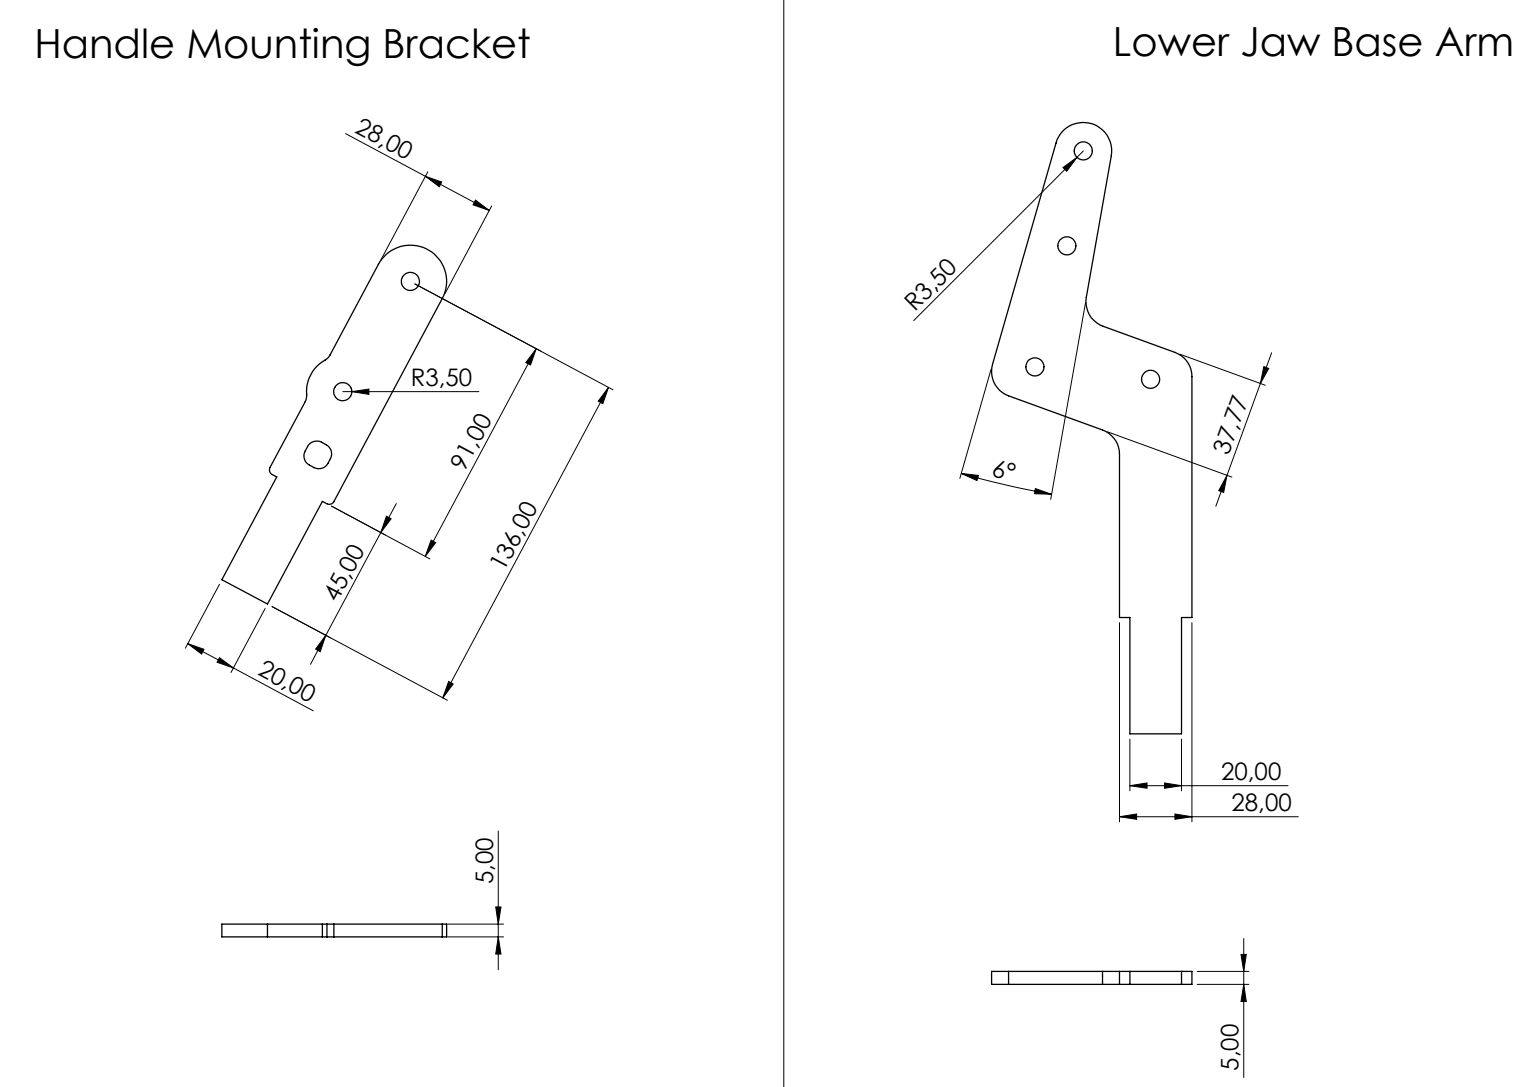
ISO-10303-21;
HEADER;
FILE_DESCRIPTION (('STEP AP214'),
    '1' );
FILE_NAME ('Lower Jaw Base Arm.step',
    '2026-10-06T08:24:18',
    ( '' ),
    ( '' ),
    'SwSTEP 2.0',
    'SolidWorks 2020',
    '' );
FILE_SCHEMA (( 'AUTOMOTIVE_DESIGN' ));
ENDSEC;

DATA;
#13=LINE ( 'NONE', #6569, #9092 ) ;
#17=UNCERTAINTY_MEASURE_WITH_UNIT (LENGTH_MEASURE( 1.000000000000000082E-05 ), #9490, 'distance_accuracy_value', 'NONE');
#20=ORIENTED_EDGE ( 'NONE', *, *, #8443, .F. ) ;
#27=EDGE_CURVE ( 'NONE', #6443, #1984, #9042, .T. ) ;
#34=EDGE_LOOP ( 'NONE', ( #2547, #9848, #2016, #7759 ) ) ;
#35=DIRECTION ( 'NONE',  ( -1.000000000000000000, 0.000000000000000000, 0.000000000000000000 ) ) ;
#41=DIRECTION ( 'NONE',  ( 0.000000000000000000, 0.000000000000000000, 1.000000000000000000 ) ) ;
#87=AXIS2_PLACEMENT_3D ( 'NONE', #9230, #1862, #35 ) ;
#93=CARTESIAN_POINT ( 'NONE',  ( 7.420201433257000545, -2.500000000000000000, -419.8948508258000061 ) ) ;
#98=DIRECTION ( 'NONE',  ( -0.9848077530122131273, 0.000000000000000000, -0.1736481776669018817 ) ) ;
#110=EDGE_LOOP ( 'NONE', ( #3310, #285 ) ) ;
#113=EDGE_CURVE ( 'NONE', #8766, #6326, #6244, .T. ) ;
#114=EDGE_CURVE ( 'NONE', #1984, #5924, #1786, .T. ) ;
#144=DIRECTION ( 'NONE',  ( 0.000000000000000000, -1.000000000000000000, 0.000000000000000000 ) ) ;
#177=CARTESIAN_POINT ( 'NONE',  ( -26.82908671702000802, -2.500000000000000000, -441.1544246730000509 ) ) ;
#178=CARTESIAN_POINT ( 'NONE',  ( 14.00000000000000000, 2.500000000000000000, -410.4979246179000256 ) ) ;
#187=AXIS2_PLACEMENT_3D ( 'NONE', #7775, #1275, #419 ) ;
#215=VERTEX_POINT ( 'NONE', #8725 ) ;
#219=DIRECTION ( 'NONE',  ( 0.9848077530122130163, 0.000000000000000000, 0.1736481776669023813 ) ) ;
#223=VERTEX_POINT ( 'NONE', #5395 ) ;
#235=EDGE_CURVE ( 'NONE', #9158, #4552, #1974, .T. ) ;
#244=CARTESIAN_POINT ( 'NONE',  ( -26.82908671702000802, -2.500000000000000000, -441.1544246730000509 ) ) ;
#285=ORIENTED_EDGE ( 'NONE', *, *, #8827, .T. ) ;
#289=VERTEX_POINT ( 'NONE', #1316 ) ;
#303=APPLICATION_CONTEXT ( 'automotive_design' ) ;
#305=DIRECTION ( 'NONE',  ( 0.000000000000000000, 1.000000000000000000, 0.000000000000000000 ) ) ;
#308=LINE ( 'NONE', #2126, #3162 ) ;
#338=LINE ( 'NONE', #980, #680 ) ;
#339=ORIENTED_EDGE ( 'NONE', *, *, #9047, .F. ) ;
#344=VERTEX_POINT ( 'NONE', #2396 ) ;
#360=CIRCLE ( 'NONE', #7394, 3.500000000000000000 ) ;
#376=CARTESIAN_POINT ( 'NONE',  ( -63.11273421720001409, 2.500000000000000000, -415.2750182148000135 ) ) ;
#377=CYLINDRICAL_SURFACE ( 'NONE', #3349, 3.500000000000003109 ) ;
#378=PLANE ( 'NONE',  #9312 ) ;
#403=ORIENTED_EDGE ( 'NONE', *, *, #6734, .T. ) ;
#419=DIRECTION ( 'NONE',  ( -0.9612616959383174509, 0.000000000000000000, -0.2756373558170044369 ) ) ;
#438=ORIENTED_EDGE ( 'NONE', *, *, #6849, .T. ) ;
#440=DIRECTION ( 'NONE',  ( 1.000000000000000000, 0.000000000000000000, 0.000000000000000000 ) ) ;
#444=EDGE_CURVE ( 'NONE', #7016, #4872, #3088, .T. ) ;
#447=CARTESIAN_POINT ( 'NONE',  ( -5.500000000000000000, 2.500000000000000000, -409.5000000000000568 ) ) ;
#478=FACE_OUTER_BOUND ( 'NONE', #9284, .T. ) ;
#480=CIRCLE ( 'NONE', #7844, 3.500000000000003109 ) ;
#494=LINE ( 'NONE', #3762, #7350 ) ;
#502=EDGE_LOOP ( 'NONE', ( #7761, #10328 ) ) ;
#506=DIRECTION ( 'NONE',  ( 1.000000000000000000, 0.000000000000000000, 0.000000000000000000 ) ) ;
#507=EDGE_CURVE ( 'NONE', #6146, #7283, #8033, .T. ) ;
#522=FILL_AREA_STYLE_COLOUR ( '', #3538 ) ;
#537=LINE ( 'NONE', #9560, #754 ) ;
#544=FACE_OUTER_BOUND ( 'NONE', #612, .T. ) ;
#549=FILL_AREA_STYLE ('',( #8596 ) ) ;
#555=CIRCLE ( 'NONE', #7588, 3.499999999999999556 ) ;
#564=CARTESIAN_POINT ( 'NONE',  ( -14.00000000000000000, 2.500000000000000000, -380.4979246178999688 ) ) ;
#580=LINE ( 'NONE', #7938, #3620 ) ;
#588=CIRCLE ( 'NONE', #7964, 3.499999999999999556 ) ;
#608=FACE_OUTER_BOUND ( 'NONE', #8794, .T. ) ;
#610=DIRECTION ( 'NONE',  ( 1.000000000000000000, 0.000000000000000000, 0.000000000000000000 ) ) ;
#612=EDGE_LOOP ( 'NONE', ( #2471, #339, #8409, #673 ) ) ;
#615=FACE_OUTER_BOUND ( 'NONE', #9397, .T. ) ;
#617=DIRECTION ( 'NONE',  ( -0.9396926207858973257, 0.000000000000000000, -0.3420201433256991330 ) ) ;
#638=ORIENTED_EDGE ( 'NONE', *, *, #1595, .F. ) ;
#657=FACE_OUTER_BOUND ( 'NONE', #6357, .T. ) ;
#658=DIRECTION ( 'NONE',  ( -1.000000000000000000, 0.000000000000000000, 0.000000000000000000 ) ) ;
#673=ORIENTED_EDGE ( 'NONE', *, *, #1413, .T. ) ;
#678=DIRECTION ( 'NONE',  ( 0.000000000000000000, 1.000000000000000000, 0.000000000000000000 ) ) ;
#680=VECTOR ( 'NONE', #1083, 1000.000000000000000 ) ;
#694=EDGE_CURVE ( 'NONE', #9461, #7519, #8991, .T. ) ;
#715=ORIENTED_EDGE ( 'NONE', *, *, #7705, .F. ) ;
#723=DIRECTION ( 'NONE',  ( 0.9848077530122130163, 0.000000000000000000, 0.1736481776669025201 ) ) ;
#731=VECTOR ( 'NONE', #6902, 1000.000000000000000 ) ;
#742=DIRECTION ( 'NONE',  ( 1.000000000000000000, 0.000000000000000000, 0.000000000000000000 ) ) ;
#754=VECTOR ( 'NONE', #1389, 1000.000000000000227 ) ;
#757=EDGE_CURVE ( 'NONE', #9634, #5121, #13, .T. ) ;
#758=DIRECTION ( 'NONE',  ( -1.000000000000000000, 0.000000000000000000, 0.000000000000000000 ) ) ;
#776=ORIENTED_EDGE ( 'NONE', *, *, #694, .F. ) ;
#816=VECTOR ( 'NONE', #6829, 1000.000000000000000 ) ;
#831=DIRECTION ( 'NONE',  ( 0.000000000000000000, -1.000000000000000000, 0.000000000000000000 ) ) ;
#853=CARTESIAN_POINT ( 'NONE',  ( 4.000000000000000000, -2.500000000000000000, -410.4979246179000256 ) ) ;
#865=VECTOR ( 'NONE', #3827, 1000.000000000000000 ) ;
#877=EDGE_LOOP ( 'NONE', ( #3684, #7845, #2714, #438 ) ) ;
#878=AXIS2_PLACEMENT_3D ( 'NONE', #2871, #7754, #8553 ) ;
#885=LINE ( 'NONE', #2614, #8061 ) ;
#886=VERTEX_POINT ( 'NONE', #9177 ) ;
#906=CARTESIAN_POINT ( 'NONE',  ( -28.01838671672000203, 2.500000000000000000, -497.7560445212000104 ) ) ;
#931=DIRECTION ( 'NONE',  ( -1.000000000000000000, 0.000000000000000000, 0.000000000000000000 ) ) ;
#940=AXIS2_PLACEMENT_3D ( 'NONE', #6757, #144, #6590 ) ;
#978=CARTESIAN_POINT ( 'NONE',  ( 14.00000000000000000, -2.500000000000000000, -410.4979246179000256 ) ) ;
#980=CARTESIAN_POINT ( 'NONE',  ( 14.00000000000000000, -2.500000000000000000, -317.5000000000000000 ) ) ;
#993=DIRECTION ( 'NONE',  ( 0.000000000000000000, -1.000000000000000000, 0.000000000000000000 ) ) ;
#995=FACE_OUTER_BOUND ( 'NONE', #6467, .T. ) ;
#997=EDGE_LOOP ( 'NONE', ( #6427, #6798, #10128, #4940 ) ) ;
#999=DIRECTION ( 'NONE',  ( 0.000000000000000000, -1.000000000000000000, 0.000000000000000000 ) ) ;
#1003=EDGE_CURVE ( 'NONE', #7519, #5811, #5243, .T. ) ;
#1024=EDGE_CURVE ( 'NONE', #5654, #10404, #308, .T. ) ;
#1027=DIRECTION ( 'NONE',  ( 0.1736481776669025201, 0.000000000000000000, -0.9848077530122130163 ) ) ;
#1031=DIRECTION ( 'NONE',  ( -1.000000000000000000, 0.000000000000000000, 0.000000000000000000 ) ) ;
#1047=DIRECTION ( 'NONE',  ( -0.9848077530122131273, 0.000000000000000000, -0.1736481776669018817 ) ) ;
#1049=CARTESIAN_POINT ( 'NONE',  ( 10.00000000000000000, -2.500000000000000000, -272.5000000000000000 ) ) ;
#1054=CARTESIAN_POINT ( 'NONE',  ( -10.00000000000000000, -2.500000000000000000, -317.5000000000000000 ) ) ;
#1065=DIRECTION ( 'NONE',  ( -0.2756373558170050475, 0.000000000000000000, 0.9612616959383172288 ) ) ;
#1079=DIRECTION ( 'NONE',  ( 0.000000000000000000, -1.000000000000000000, 0.000000000000000000 ) ) ;
#1083=DIRECTION ( 'NONE',  ( 0.000000000000000000, 1.000000000000000000, 0.000000000000000000 ) ) ;
#1084=EDGE_CURVE ( 'NONE', #6576, #215, #8309, .T. ) ;
#1103=ORIENTED_EDGE ( 'NONE', *, *, #7129, .T. ) ;
#1111=AXIS2_PLACEMENT_3D ( 'NONE', #8004, #8802, #4672 ) ;
#1143=CARTESIAN_POINT ( 'NONE',  ( 14.00000000000000000, -2.500000000000000000, -317.5000000000000000 ) ) ;
#1151=DIRECTION ( 'NONE',  ( 0.000000000000000000, 1.000000000000000000, 0.000000000000000000 ) ) ;
#1162=CIRCLE ( 'NONE', #3220, 11.00000000000000000 ) ;
#1175=LINE ( 'NONE', #8742, #10006 ) ;
#1185=DIRECTION ( 'NONE',  ( 0.9848077530122130163, 0.000000000000000000, 0.1736481776669023813 ) ) ;
#1188=EDGE_LOOP ( 'NONE', ( #2072, #8240, #8227, #5008 ) ) ;
#1194=AXIS2_PLACEMENT_3D ( 'NONE', #4119, #993, #6644 ) ;
#1201=ORIENTED_EDGE ( 'NONE', *, *, #1003, .T. ) ;
#1215=LINE ( 'NONE', #2785, #8659 ) ;
#1220=EDGE_LOOP ( 'NONE', ( #1727, #6254 ) ) ;
#1223=EDGE_CURVE ( 'NONE', #8790, #6146, #8438, .T. ) ;
#1229=LINE ( 'NONE', #6992, #2985 ) ;
#1233=AXIS2_PLACEMENT_3D ( 'NONE', #8007, #6501, #4787 ) ;
#1239=ADVANCED_FACE ( 'NONE', ( #4414 ), #6790, .T. ) ;
#1245=DIRECTION ( 'NONE',  ( 0.000000000000000000, 1.000000000000000000, 0.000000000000000000 ) ) ;
#1262=CARTESIAN_POINT ( 'NONE',  ( -37.87192209818999800, 2.500000000000000000, -461.0868123482000556 ) ) ;
#1273=ORIENTED_EDGE ( 'NONE', *, *, #1410, .F. ) ;
#1275=DIRECTION ( 'NONE',  ( 0.000000000000000000, 1.000000000000000000, 0.000000000000000000 ) ) ;
#1277=ADVANCED_FACE ( 'NONE', ( #8390, #4462, #9365, #4264, #6943 ), #4313, .F. ) ;
#1285=CARTESIAN_POINT ( 'NONE',  ( 4.000000000000000000, 2.656480000000000175, -410.4979246179000256 ) ) ;
#1290=CARTESIAN_POINT ( 'NONE',  ( 7.420201433257000545, 2.500000000000000000, -419.8948508258000061 ) ) ;
#1299=SURFACE_STYLE_USAGE ( .BOTH. , #10379 ) ;
#1316=CARTESIAN_POINT ( 'NONE',  ( 14.00000000000000000, 2.500000000000000000, -317.5000000000000000 ) ) ;
#1322=VERTEX_POINT ( 'NONE', #178 ) ;
#1324=AXIS2_PLACEMENT_3D ( 'NONE', #4265, #1079, #7534 ) ;
#1358=PLANE ( 'NONE',  #3824 ) ;
#1359=EDGE_LOOP ( 'NONE', ( #1930, #10581, #4963, #3339 ) ) ;
#1381=COLOUR_RGB ( '', 0.09019608, 0.27058824, 0.51372549) ;
#1385=DIRECTION ( 'NONE',  ( 0.000000000000000000, 1.000000000000000000, 0.000000000000000000 ) ) ;
#1389=DIRECTION ( 'NONE',  ( 0.9396926207858972147, 0.000000000000000000, 0.3420201433256990775 ) ) ;
#1405=PRESENTATION_STYLE_ASSIGNMENT (( #1299 ) ) ;
#1410=EDGE_CURVE ( 'NONE', #1779, #9634, #8644, .T. ) ;
#1413=EDGE_CURVE ( 'NONE', #9766, #8632, #588, .T. ) ;
#1437=ORIENTED_EDGE ( 'NONE', *, *, #3941, .F. ) ;
#1447=ORIENTED_EDGE ( 'NONE', *, *, #3836, .F. ) ;
#1465=DIRECTION ( 'NONE',  ( 0.000000000000000000, -1.000000000000000000, 0.000000000000000000 ) ) ;
#1474=DIRECTION ( 'NONE',  ( 0.000000000000000000, 0.000000000000000000, -1.000000000000000000 ) ) ;
#1479=ORIENTED_EDGE ( 'NONE', *, *, #6849, .F. ) ;
#1496=FACE_OUTER_BOUND ( 'NONE', #9347, .T. ) ;
#1510=VECTOR ( 'NONE', #8979, 1000.000000000000000 ) ;
#1511=LINE ( 'NONE', #4035, #8370 ) ;
#1517=CYLINDRICAL_SURFACE ( 'NONE', #2762, 3.499999999999999556 ) ;
#1529=LINE ( 'NONE', #564, #1934 ) ;
#1533=CARTESIAN_POINT ( 'NONE',  ( -30.87192209819000155, 2.500000000000000000, -461.0868123482000556 ) ) ;
#1539=VECTOR ( 'NONE', #4099, 1000.000000000000000 ) ;
#1554=CARTESIAN_POINT ( 'NONE',  ( -20.57979856674000629, -2.500000000000000000, -389.8948508258000061 ) ) ;
#1572=CARTESIAN_POINT ( 'NONE',  ( 14.00000000000000000, 2.500000000000000000, -410.4979246179000256 ) ) ;
#1595=EDGE_CURVE ( 'NONE', #5654, #6416, #2475, .T. ) ;
#1615=ORIENTED_EDGE ( 'NONE', *, *, #1024, .T. ) ;
#1621=CIRCLE ( 'NONE', #7626, 3.499999999999999556 ) ;
#1647=EDGE_LOOP ( 'NONE', ( #8599, #7824, #2420, #5607 ) ) ;
#1650=ORIENTED_EDGE ( 'NONE', *, *, #2610, .F. ) ;
#1654=DIRECTION ( 'NONE',  ( 0.000000000000000000, -1.000000000000000000, 0.000000000000000000 ) ) ;
#1667=ADVANCED_FACE ( 'NONE', ( #2269 ), #5535, .T. ) ;
#1673=CARTESIAN_POINT ( 'NONE',  ( -20.57979856674000629, 2.500000000000000000, -389.8948508258000061 ) ) ;
#1684=AXIS2_PLACEMENT_3D ( 'NONE', #10257, #2846, #2193 ) ;
#1695=MANIFOLD_SOLID_BREP ( 'Stock-MAS-686-1', #6776 ) ;
#1707=CYLINDRICAL_SURFACE ( 'NONE', #5477, 10.00000000000000000 ) ;
#1727=ORIENTED_EDGE ( 'NONE', *, *, #8494, .F. ) ;
#1736=DIRECTION ( 'NONE',  ( 0.000000000000000000, -1.000000000000000000, 0.000000000000000000 ) ) ;
#1747=CARTESIAN_POINT ( 'NONE',  ( -37.87192209818999800, -2.500000000000000000, -461.0868123482000556 ) ) ;
#1752=EDGE_CURVE ( 'NONE', #1322, #1779, #6013, .T. ) ;
#1764=LINE ( 'NONE', #5952, #10510 ) ;
#1779=VERTEX_POINT ( 'NONE', #5592 ) ;
#1786=LINE ( 'NONE', #5056, #7970 ) ;
#1801=ADVANCED_FACE ( 'NONE', ( #8069 ), #1517, .F. ) ;
#1807=EDGE_CURVE ( 'NONE', #6443, #6958, #3284, .T. ) ;
#1827=EDGE_LOOP ( 'NONE', ( #5391, #2707, #3495, #4698 ) ) ;
#1853=ORIENTED_EDGE ( 'NONE', *, *, #2590, .F. ) ;
#1862=DIRECTION ( 'NONE',  ( 0.000000000000000000, -1.000000000000000000, 0.000000000000000000 ) ) ;
#1872=DIRECTION ( 'NONE',  ( 0.000000000000000000, 1.000000000000000000, 0.000000000000000000 ) ) ;
#1891=EDGE_CURVE ( 'NONE', #1322, #2247, #9793, .T. ) ;
#1901=AXIS2_PLACEMENT_3D ( 'NONE', #2432, #3345, #5855 ) ;
#1903=ORIENTED_EDGE ( 'NONE', *, *, #444, .T. ) ;
#1918=LINE ( 'NONE', #1054, #6408 ) ;
#1924=PRODUCT ( 'Lower Jaw Base Arm', 'Lower Jaw Base Arm', '', ( #5587 ) ) ;
#1930=ORIENTED_EDGE ( 'NONE', *, *, #3836, .T. ) ;
#1934=VECTOR ( 'NONE', #3840, 1000.000000000000000 ) ;
#1940=EDGE_CURVE ( 'NONE', #223, #8573, #5502, .T. ) ;
#1973=DIRECTION ( 'NONE',  ( 0.000000000000000000, -1.000000000000000000, 0.000000000000000000 ) ) ;
#1974=LINE ( 'NONE', #1262, #10038 ) ;
#1976=CIRCLE ( 'NONE', #6248, 3.500000000000003109 ) ;
#1982=CARTESIAN_POINT ( 'NONE',  ( 14.00000000000000000, -2.500000000000000000, -417.5000000000000000 ) ) ;
#1984=VERTEX_POINT ( 'NONE', #5436 ) ;
#1993=DIRECTION ( 'NONE',  ( 0.000000000000000000, -1.000000000000000000, 0.000000000000000000 ) ) ;
#2016=ORIENTED_EDGE ( 'NONE', *, *, #4776, .F. ) ;
#2036=DIRECTION ( 'NONE',  ( -1.000000000000000000, 0.000000000000000000, 0.000000000000000000 ) ) ;
#2068=EDGE_CURVE ( 'NONE', #7519, #2769, #7910, .T. ) ;
#2072=ORIENTED_EDGE ( 'NONE', *, *, #9179, .F. ) ;
#2078=ADVANCED_FACE ( 'NONE', ( #4696, #6298, #7972, #6962, #615 ), #7067, .T. ) ;
#2079=LINE ( 'NONE', #9343, #6392 ) ;
#2108=VECTOR ( 'NONE', #1151, 1000.000000000000000 ) ;
#2111=DIRECTION ( 'NONE',  ( 0.000000000000000000, 0.000000000000000000, -1.000000000000000000 ) ) ;
#2120=ADVANCED_FACE ( 'NONE', ( #5600 ), #4803, .F. ) ;
#2126=CARTESIAN_POINT ( 'NONE',  ( 1.499999999999999556, 2.500000000000000000, -409.5000000000000568 ) ) ;
#2134=FACE_OUTER_BOUND ( 'NONE', #8477, .T. ) ;
#2148=AXIS2_PLACEMENT_3D ( 'NONE', #1982, #4493, #10142 ) ;
#2158=CYLINDRICAL_SURFACE ( 'NONE', #9318, 3.500000000000003109 ) ;
#2162=CARTESIAN_POINT ( 'NONE',  ( -31.51838671672000558, -2.500000000000000000, -497.7560445212000104 ) ) ;
#2173=AXIS2_PLACEMENT_3D ( 'NONE', #6893, #10160, #9209 ) ;
#2174=CARTESIAN_POINT ( 'NONE',  ( -28.28616793536999907, -2.500000000000000000, -432.8909064497000259 ) ) ;
#2193=DIRECTION ( 'NONE',  ( 0.000000000000000000, -1.000000000000000000, 0.000000000000000000 ) ) ;
#2217=( LENGTH_UNIT ( ) NAMED_UNIT ( * ) SI_UNIT ( .MILLI., .METRE. ) );
#2227=FACE_OUTER_BOUND ( 'NONE', #997, .T. ) ;
#2234=DIRECTION ( 'NONE',  ( 0.000000000000000000, -1.000000000000000000, 0.000000000000000000 ) ) ;
#2246=ADVANCED_FACE ( 'NONE', ( #8391 ), #6842, .F. ) ;
#2247=VERTEX_POINT ( 'NONE', #978 ) ;
#2259=PLANE ( 'NONE',  #5785 ) ;
#2269=FACE_OUTER_BOUND ( 'NONE', #4438, .T. ) ;
#2271=ORIENTED_EDGE ( 'NONE', *, *, #694, .T. ) ;
#2281=ORIENTED_EDGE ( 'NONE', *, *, #757, .F. ) ;
#2285=ORIENTED_EDGE ( 'NONE', *, *, #235, .F. ) ;
#2317=EDGE_CURVE ( 'NONE', #6229, #4674, #6126, .T. ) ;
#2324=CARTESIAN_POINT ( 'NONE',  ( -26.82908671702000802, -2.500000000000000000, -441.1544246730000509 ) ) ;
#2337=CARTESIAN_POINT ( 'NONE',  ( 10.00000000000000000, 2.500000000000000000, -272.5000000000000000 ) ) ;
#2351=ORIENTED_EDGE ( 'NONE', *, *, #5085, .T. ) ;
#2358=CYLINDRICAL_SURFACE ( 'NONE', #6355, 11.00000000000000000 ) ;
#2389=EDGE_LOOP ( 'NONE', ( #6696, #4034, #7884, #9897 ) ) ;
#2396=CARTESIAN_POINT ( 'NONE',  ( -43.24071243418999444, -2.500000000000000000, -414.3237589990000629 ) ) ;
#2418=LINE ( 'NONE', #6552, #7791 ) ;
#2419=CIRCLE ( 'NONE', #1901, 10.00000000000000533 ) ;
#2420=ORIENTED_EDGE ( 'NONE', *, *, #9961, .T. ) ;
#2432=CARTESIAN_POINT ( 'NONE',  ( -16.98100918689000238, 2.500000000000000000, -439.4179428962999623 ) ) ;
#2447=CARTESIAN_POINT ( 'NONE',  ( -53.50011725782000127, -2.500000000000000000, -412.5186446566000313 ) ) ;
#2463=EDGE_CURVE ( 'NONE', #1779, #3477, #1511, .T. ) ;
#2471=ORIENTED_EDGE ( 'NONE', *, *, #10174, .F. ) ;
#2472=DIRECTION ( 'NONE',  ( 0.000000000000000000, -1.000000000000000000, 0.000000000000000000 ) ) ;
#2475=CIRCLE ( 'NONE', #9348, 3.500000000000000000 ) ;
#2504=ADVANCED_FACE ( 'NONE', ( #4841 ), #2259, .T. ) ;
#2512=ORIENTED_EDGE ( 'NONE', *, *, #2068, .T. ) ;
#2516=CARTESIAN_POINT ( 'NONE',  ( 10.00000000000000000, 2.500000000000000000, -317.5000000000000000 ) ) ;
#2526=EDGE_LOOP ( 'NONE', ( #7414, #638, #1615, #1103 ) ) ;
#2534=DIRECTION ( 'NONE',  ( 0.000000000000000000, -1.000000000000000000, 0.000000000000000000 ) ) ;
#2542=EDGE_CURVE ( 'NONE', #4674, #344, #480, .T. ) ;
#2547=ORIENTED_EDGE ( 'NONE', *, *, #2556, .T. ) ;
#2551=ORIENTED_EDGE ( 'NONE', *, *, #9062, .T. ) ;
#2556=EDGE_CURVE ( 'NONE', #9461, #6326, #6334, .T. ) ;
#2576=ORIENTED_EDGE ( 'NONE', *, *, #6072, .T. ) ;
#2589=DIRECTION ( 'NONE',  ( 1.000000000000000000, 0.000000000000000000, 0.000000000000000000 ) ) ;
#2590=EDGE_CURVE ( 'NONE', #8773, #8790, #6665, .T. ) ;
#2594=DIRECTION ( 'NONE',  ( 0.3420201433256988555, 0.000000000000000000, -0.9396926207858975477 ) ) ;
#2600=PRODUCT_DEFINITION_CONTEXT ( 'detailed design', #303, 'design' ) ;
#2610=EDGE_CURVE ( 'NONE', #5924, #4480, #1162, .T. ) ;
#2614=CARTESIAN_POINT ( 'NONE',  ( -56.92031869107000119, 2.500000000000000000, -403.1217184488000385 ) ) ;
#2633=ORIENTED_EDGE ( 'NONE', *, *, #1410, .T. ) ;
#2636=ORIENTED_EDGE ( 'NONE', *, *, #3707, .T. ) ;
#2679=EDGE_CURVE ( 'NONE', #9887, #7283, #8427, .T. ) ;
#2705=UNCERTAINTY_MEASURE_WITH_UNIT (LENGTH_MEASURE( 1.000000000000000082E-05 ), #4488, 'distance_accuracy_value', 'NONE');
#2706=LINE ( 'NONE', #4318, #5817 ) ;
#2707=ORIENTED_EDGE ( 'NONE', *, *, #6734, .F. ) ;
#2714=ORIENTED_EDGE ( 'NONE', *, *, #235, .T. ) ;
#2762=AXIS2_PLACEMENT_3D ( 'NONE', #9901, #4149, #8225 ) ;
#2769=VERTEX_POINT ( 'NONE', #4609 ) ;
#2774=ORIENTED_EDGE ( 'NONE', *, *, #1413, .F. ) ;
#2785=CARTESIAN_POINT ( 'NONE',  ( -10.00000000000000000, 2.500000000000000000, -317.5000000000000000 ) ) ;
#2814=ORIENTED_EDGE ( 'NONE', *, *, #3455, .T. ) ;
#2817=AXIS2_PLACEMENT_3D ( 'NONE', #8634, #3966, #3161 ) ;
#2818=LINE ( 'NONE', #6093, #4530 ) ;
#2819=ORIENTED_EDGE ( 'NONE', *, *, #2463, .F. ) ;
#2828=ADVANCED_FACE ( 'NONE', ( #478 ), #6275, .T. ) ;
#2846=DIRECTION ( 'NONE',  ( 0.000000000000000000, 0.000000000000000000, 1.000000000000000000 ) ) ;
#2851=CARTESIAN_POINT ( 'NONE',  ( -17.01838671672000203, -2.500000000000000000, -497.7560445212000104 ) ) ;
#2871=CARTESIAN_POINT ( 'NONE',  ( -28.01838671672000203, -2.500000000000000000, -497.7560445212000104 ) ) ;
#2872=EDGE_CURVE ( 'NONE', #3553, #344, #4406, .T. ) ;
#2889=EDGE_LOOP ( 'NONE', ( #8940, #2351, #1650, #7221 ) ) ;
#2901=DIRECTION ( 'NONE',  ( 0.000000000000000000, 1.000000000000000000, 0.000000000000000000 ) ) ;
#2905=DIRECTION ( 'NONE',  ( 0.000000000000000000, -1.000000000000000000, 0.000000000000000000 ) ) ;
#2916=CARTESIAN_POINT ( 'NONE',  ( -24.51838671671999847, 2.500000000000000000, -497.7560445212000104 ) ) ;
#2944=CIRCLE ( 'NONE', #1233, 10.00000000000000000 ) ;
#2958=AXIS2_PLACEMENT_3D ( 'NONE', #7944, #9505, #7095 ) ;
#2959=ORIENTED_EDGE ( 'NONE', *, *, #7600, .T. ) ;
#2977=ORIENTED_EDGE ( 'NONE', *, *, #3168, .F. ) ;
#2984=ORIENTED_EDGE ( 'NONE', *, *, #3202, .T. ) ;
#2985=VECTOR ( 'NONE', #2901, 1000.000000000000000 ) ;
#2993=ORIENTED_EDGE ( 'NONE', *, *, #7129, .F. ) ;
#3012=DIRECTION ( 'NONE',  ( -1.000000000000000000, 0.000000000000000000, 0.000000000000000000 ) ) ;
#3019=SURFACE_STYLE_FILL_AREA ( #549 ) ;
#3025=DIRECTION ( 'NONE',  ( 1.000000000000000000, 0.000000000000000000, 0.000000000000000000 ) ) ;
#3027=ORIENTED_EDGE ( 'NONE', *, *, #4829, .F. ) ;
#3088=LINE ( 'NONE', #1533, #9854 ) ;
#3100=DIRECTION ( 'NONE',  ( 0.000000000000000000, 1.000000000000000000, 0.000000000000000000 ) ) ;
#3161=DIRECTION ( 'NONE',  ( 1.000000000000000000, 0.000000000000000000, 0.000000000000000000 ) ) ;
#3162=VECTOR ( 'NONE', #1973, 1000.000000000000000 ) ;
#3168=EDGE_CURVE ( 'NONE', #4480, #5049, #3226, .T. ) ;
#3174=DIRECTION ( 'NONE',  ( -1.000000000000000000, 0.000000000000000000, 0.000000000000000000 ) ) ;
#3180=PLANE ( 'NONE',  #9106 ) ;
#3197=ORIENTED_EDGE ( 'NONE', *, *, #1024, .F. ) ;
#3202=EDGE_CURVE ( 'NONE', #7283, #289, #494, .T. ) ;
#3204=ADVANCED_FACE ( 'NONE', ( #544 ), #2158, .F. ) ;
#3220=AXIS2_PLACEMENT_3D ( 'NONE', #9198, #7573, #219 ) ;
#3226=CIRCLE ( 'NONE', #9243, 11.00000000000000000 ) ;
#3231=CARTESIAN_POINT ( 'NONE',  ( -28.01838671672000203, -2.500000000000000000, -497.7560445212000104 ) ) ;
#3254=AXIS2_PLACEMENT_3D ( 'NONE', #4212, #4371, #1031 ) ;
#3284=LINE ( 'NONE', #2324, #7395 ) ;
#3310=ORIENTED_EDGE ( 'NONE', *, *, #3941, .T. ) ;
#3316=CARTESIAN_POINT ( 'NONE',  ( -31.51838671672000558, 2.500000000000000000, -497.7560445212000104 ) ) ;
#3322=CARTESIAN_POINT ( 'NONE',  ( -24.00000000000000000, -2.633704000000000267, -380.4979246178999688 ) ) ;
#3339=ORIENTED_EDGE ( 'NONE', *, *, #10161, .T. ) ;
#3345=DIRECTION ( 'NONE',  ( 0.000000000000000000, -1.000000000000000000, 0.000000000000000000 ) ) ;
#3349=AXIS2_PLACEMENT_3D ( 'NONE', #4563, #1993, #7735 ) ;
#3362=STYLED_ITEM ( 'NONE', ( #7988 ), #3778 ) ;
#3387=EDGE_LOOP ( 'NONE', ( #2271, #1201, #9015, #8550 ) ) ;
#3397=ADVANCED_FACE ( 'NONE', ( #3807 ), #7040, .F. ) ;
#3435=DIRECTION ( 'NONE',  ( -1.000000000000000000, 0.000000000000000000, 0.000000000000000000 ) ) ;
#3436=ORIENTED_EDGE ( 'NONE', *, *, #9040, .F. ) ;
#3442=AXIS2_PLACEMENT_3D ( 'NONE', #5108, #3860, #2036 ) ;
#3455=EDGE_CURVE ( 'NONE', #8573, #5049, #1175, .T. ) ;
#3470=DIRECTION ( 'NONE',  ( 0.000000000000000000, 1.000000000000000000, 0.000000000000000000 ) ) ;
#3477=VERTEX_POINT ( 'NONE', #3649 ) ;
#3495=ORIENTED_EDGE ( 'NONE', *, *, #9062, .F. ) ;
#3506=CARTESIAN_POINT ( 'NONE',  ( -34.37192209818999800, -2.500000000000000000, -461.0868123482000556 ) ) ;
#3518=PLANE ( 'NONE',  #8100 ) ;
#3538=COLOUR_RGB ( '', 0.09019608, 0.27058824, 0.51372549) ;
#3550=CARTESIAN_POINT ( 'NONE',  ( 10.00000000000000000, 2.500000000000000000, -272.5000000000000000 ) ) ;
#3553=VERTEX_POINT ( 'NONE', #5734 ) ;
#3574=VECTOR ( 'NONE', #4453, 1000.000000000000000 ) ;
#3581=CARTESIAN_POINT ( 'NONE',  ( -24.51838671671999847, -2.500000000000000000, -497.7560445212000104 ) ) ;
#3582=VERTEX_POINT ( 'NONE', #1554 ) ;
#3620=VECTOR ( 'NONE', #9401, 1000.000000000000000 ) ;
#3623=ORIENTED_EDGE ( 'NONE', *, *, #1940, .T. ) ;
#3635=CARTESIAN_POINT ( 'NONE',  ( -56.92031869107000119, 2.500000000000000000, -403.1217184488000385 ) ) ;
#3639=DIRECTION ( 'NONE',  ( 0.9396926207858972147, 0.000000000000000000, 0.3420201433256990775 ) ) ;
#3647=CIRCLE ( 'NONE', #9146, 3.499999999999999556 ) ;
#3649=CARTESIAN_POINT ( 'NONE',  ( -20.40121062015000319, 2.500000000000000000, -430.0210166885000262 ) ) ;
#3657=DIRECTION ( 'NONE',  ( 1.000000000000000000, 0.000000000000000000, 0.000000000000000000 ) ) ;
#3670=AXIS2_PLACEMENT_3D ( 'NONE', #8121, #6401, #758 ) ;
#3672=AXIS2_PLACEMENT_3D ( 'NONE', #6674, #9953, #2594 ) ;
#3684=ORIENTED_EDGE ( 'NONE', *, *, #444, .F. ) ;
#3707=EDGE_CURVE ( 'NONE', #6146, #4332, #5195, .T. ) ;
#3749=CARTESIAN_POINT ( 'NONE',  ( -10.00000000000000000, -2.500000000000000000, -317.5000000000000000 ) ) ;
#3755=FACE_OUTER_BOUND ( 'NONE', #1188, .T. ) ;
#3762=CARTESIAN_POINT ( 'NONE',  ( 10.00000000000000000, 2.500000000000000000, -317.5000000000000000 ) ) ;
#3778=ADVANCED_BREP_SHAPE_REPRESENTATION ( '', ( #1695, #2817 ), #7476 ) ;
#3785=ORIENTED_EDGE ( 'NONE', *, *, #4128, .T. ) ;
#3803=ADVANCED_FACE ( 'NONE', ( #5891 ), #9932, .F. ) ;
#3806=PLANE ( 'NONE',  #6070 ) ;
#3807=FACE_OUTER_BOUND ( 'NONE', #10083, .T. ) ;
#3820=DIRECTION ( 'NONE',  ( 0.000000000000000000, -1.000000000000000000, 0.000000000000000000 ) ) ;
#3823=CARTESIAN_POINT ( 'NONE',  ( -16.98100918689000238, -2.500000000000000000, -439.4179428962999623 ) ) ;
#3824=AXIS2_PLACEMENT_3D ( 'NONE', #4641, #9584, #617 ) ;
#3826=DIRECTION ( 'NONE',  ( -0.3420201433256988555, 0.000000000000000000, 0.9396926207858975477 ) ) ;
#3827=DIRECTION ( 'NONE',  ( 0.000000000000000000, -1.000000000000000000, 0.000000000000000000 ) ) ;
#3833=CARTESIAN_POINT ( 'NONE',  ( 14.00000000000000000, 2.500000000000000000, -317.5000000000000000 ) ) ;
#3836=EDGE_CURVE ( 'NONE', #8773, #4852, #1764, .T. ) ;
#3839=ORIENTED_EDGE ( 'NONE', *, *, #2317, .T. ) ;
#3840=DIRECTION ( 'NONE',  ( 0.000000000000000000, 0.000000000000000000, 1.000000000000000000 ) ) ;
#3844=EDGE_CURVE ( 'NONE', #10456, #8766, #2079, .T. ) ;
#3848=VECTOR ( 'NONE', #3875, 1000.000000000000000 ) ;
#3860=DIRECTION ( 'NONE',  ( 0.000000000000000000, -1.000000000000000000, 0.000000000000000000 ) ) ;
#3870=DIRECTION ( 'NONE',  ( -0.2756373558170050475, 0.000000000000000000, 0.9612616959383172288 ) ) ;
#3875=DIRECTION ( 'NONE',  ( 0.000000000000000000, -1.000000000000000000, 0.000000000000000000 ) ) ;
#3931=CARTESIAN_POINT ( 'NONE',  ( 10.00000000000000000, -2.500000000000000000, -272.5000000000000000 ) ) ;
#3941=EDGE_CURVE ( 'NONE', #7016, #9158, #3647, .T. ) ;
#3966=DIRECTION ( 'NONE',  ( 0.000000000000000000, 0.000000000000000000, 1.000000000000000000 ) ) ;
#3999=CARTESIAN_POINT ( 'NONE',  ( -10.00000000000000000, 2.500000000000000000, -272.5000000000000000 ) ) ;
#4002=CARTESIAN_POINT ( 'NONE',  ( 10.00000000000000000, -2.500000000000000000, -317.5000000000000000 ) ) ;
#4034=ORIENTED_EDGE ( 'NONE', *, *, #6814, .F. ) ;
#4035=CARTESIAN_POINT ( 'NONE',  ( 7.420201433257000545, 2.500000000000000000, -419.8948508258000061 ) ) ;
#4052=EDGE_CURVE ( 'NONE', #6958, #5924, #5282, .T. ) ;
#4058=ORIENTED_EDGE ( 'NONE', *, *, #2463, .T. ) ;
#4064=AXIS2_PLACEMENT_3D ( 'NONE', #5165, #6733, #3657 ) ;
#4099=DIRECTION ( 'NONE',  ( 0.000000000000000000, 0.000000000000000000, 1.000000000000000000 ) ) ;
#4110=DIRECTION ( 'NONE',  ( -0.3420201433256988555, 0.000000000000000000, 0.9396926207858975477 ) ) ;
#4119=CARTESIAN_POINT ( 'NONE',  ( -46.74071243419000155, -2.500000000000000000, -414.3237589990000629 ) ) ;
#4120=ORIENTED_EDGE ( 'NONE', *, *, #6677, .T. ) ;
#4122=ADVANCED_FACE ( 'NONE', ( #4755 ), #1358, .T. ) ;
#4128=EDGE_CURVE ( 'NONE', #289, #1322, #10491, .T. ) ;
#4129=DIRECTION ( 'NONE',  ( 1.000000000000000000, 0.000000000000000000, 0.000000000000000000 ) ) ;
#4138=STYLED_ITEM ( 'NONE', ( #1405 ), #1695 ) ;
#4149=DIRECTION ( 'NONE',  ( 0.000000000000000000, -1.000000000000000000, 0.000000000000000000 ) ) ;
#4212=CARTESIAN_POINT ( 'NONE',  ( -2.000000000000000000, -2.500000000000000000, -409.5000000000000568 ) ) ;
#4218=ORIENTED_EDGE ( 'NONE', *, *, #6330, .T. ) ;
#4248=ORIENTED_EDGE ( 'NONE', *, *, #2542, .T. ) ;
#4263=VECTOR ( 'NONE', #6948, 1000.000000000000000 ) ;
#4264=FACE_BOUND ( 'NONE', #9002, .T. ) ;
#4265=CARTESIAN_POINT ( 'NONE',  ( -34.37192209818999800, 2.500000000000000000, -461.0868123482000556 ) ) ;
#4290=CIRCLE ( 'NONE', #3254, 3.499999999999999556 ) ;
#4313=PLANE ( 'NONE',  #2173 ) ;
#4318=CARTESIAN_POINT ( 'NONE',  ( -63.11273421720001409, 2.500000000000000000, -415.2750182148000135 ) ) ;
#4322=LINE ( 'NONE', #10068, #7974 ) ;
#4332=VERTEX_POINT ( 'NONE', #9296 ) ;
#4341=VECTOR ( 'NONE', #6820, 1000.000000000000000 ) ;
#4354=CARTESIAN_POINT ( 'NONE',  ( -10.00000000000000000, -2.500000000000000000, -272.5000000000000000 ) ) ;
#4365=CARTESIAN_POINT ( 'NONE',  ( 10.00000000000000000, -2.500000000000000000, -272.5000000000000000 ) ) ;
#4371=DIRECTION ( 'NONE',  ( 0.000000000000000000, -1.000000000000000000, 0.000000000000000000 ) ) ;
#4376=CARTESIAN_POINT ( 'NONE',  ( -5.500000000000000000, 2.500000000000000000, -409.5000000000000568 ) ) ;
#4395=MECHANICAL_DESIGN_GEOMETRIC_PRESENTATION_REPRESENTATION('',(#3362),#9367);
#4406=LINE ( 'NONE', #6164, #3574 ) ;
#4412=PRODUCT_DEFINITION_SHAPE ( 'NONE', 'NONE',  #8229 ) ;
#4414=FACE_OUTER_BOUND ( 'NONE', #2889, .T. ) ;
#4438=EDGE_LOOP ( 'NONE', ( #20, #10120, #2959, #9597 ) ) ;
#4446=PLANE ( 'NONE',  #2148 ) ;
#4453=DIRECTION ( 'NONE',  ( 0.000000000000000000, -1.000000000000000000, 0.000000000000000000 ) ) ;
#4462=FACE_BOUND ( 'NONE', #1220, .T. ) ;
#4471=EDGE_LOOP ( 'NONE', ( #4719, #10570, #9184, #1853, #5866, #9685, #776, #5992, #3436, #4965, #7187, #9319, #9698, #9572, #6662, #2281, #7184 ) ) ;
#4474=CARTESIAN_POINT ( 'NONE',  ( -14.00000000000000000, -2.500000000000000000, -317.5000000000000000 ) ) ;
#4480=VERTEX_POINT ( 'NONE', #8087 ) ;
#4481=CARTESIAN_POINT ( 'NONE',  ( -10.00000000000000000, -2.500000000000000000, -317.5000000000000000 ) ) ;
#4484=DIRECTION ( 'NONE',  ( 0.000000000000000000, 1.000000000000000000, 0.000000000000000000 ) ) ;
#4488=( LENGTH_UNIT ( ) NAMED_UNIT ( * ) SI_UNIT ( .MILLI., .METRE. ) );
#4492=AXIS2_PLACEMENT_3D ( 'NONE', #906, #7413, #4991 ) ;
#4493=DIRECTION ( 'NONE',  ( 0.3420201433256991330, 0.000000000000000000, -0.9396926207858973257 ) ) ;
#4495=ORIENTED_EDGE ( 'NONE', *, *, #2679, .F. ) ;
#4522=LINE ( 'NONE', #447, #865 ) ;
#4523=ORIENTED_EDGE ( 'NONE', *, *, #6931, .T. ) ;
#4530=VECTOR ( 'NONE', #3470, 1000.000000000000000 ) ;
#4536=ORIENTED_EDGE ( 'NONE', *, *, #6814, .T. ) ;
#4552=VERTEX_POINT ( 'NONE', #1747 ) ;
#4563=CARTESIAN_POINT ( 'NONE',  ( -34.37192209818999800, 2.500000000000000000, -461.0868123482000556 ) ) ;
#4569=DIRECTION ( 'NONE',  ( 1.000000000000000000, 0.000000000000000000, 0.000000000000000000 ) ) ;
#4586=AXIS2_PLACEMENT_3D ( 'NONE', #8881, #4752, #8829 ) ;
#4609=CARTESIAN_POINT ( 'NONE',  ( -10.00000000000000000, -2.500000000000000000, -317.5000000000000000 ) ) ;
#4631=DIRECTION ( 'NONE',  ( 0.000000000000000000, 1.000000000000000000, 0.000000000000000000 ) ) ;
#4641=CARTESIAN_POINT ( 'NONE',  ( -65.68309414322000350, -2.500000000000000000, -406.3111078829000462 ) ) ;
#4642=ORIENTED_EDGE ( 'NONE', *, *, #3168, .T. ) ;
#4672=DIRECTION ( 'NONE',  ( 0.9848077530122130163, 0.000000000000000000, 0.1736481776669023813 ) ) ;
#4674=VERTEX_POINT ( 'NONE', #7289 ) ;
#4686=PLANE ( 'NONE',  #9440 ) ;
#4696=FACE_BOUND ( 'NONE', #9134, .T. ) ;
#4698=ORIENTED_EDGE ( 'NONE', *, *, #8571, .F. ) ;
#4719=ORIENTED_EDGE ( 'NONE', *, *, #9961, .F. ) ;
#4752=DIRECTION ( 'NONE',  ( 0.000000000000000000, -1.000000000000000000, 0.000000000000000000 ) ) ;
#4755=FACE_OUTER_BOUND ( 'NONE', #9249, .T. ) ;
#4772=VECTOR ( 'NONE', #8271, 1000.000000000000000 ) ;
#4776=EDGE_CURVE ( 'NONE', #3582, #8766, #2818, .T. ) ;
#4787=DIRECTION ( 'NONE',  ( 1.000000000000000000, 0.000000000000000000, 0.000000000000000000 ) ) ;
#4790=DIRECTION ( 'NONE',  ( 0.000000000000000000, -1.000000000000000000, 0.000000000000000000 ) ) ;
#4803=CYLINDRICAL_SURFACE ( 'NONE', #4586, 3.500000000000003109 ) ;
#4829=EDGE_CURVE ( 'NONE', #8632, #9766, #1976, .T. ) ;
#4841=FACE_OUTER_BOUND ( 'NONE', #6864, .T. ) ;
#4852=VERTEX_POINT ( 'NONE', #10428 ) ;
#4872=VERTEX_POINT ( 'NONE', #8176 ) ;
#4898=DIRECTION ( 'NONE',  ( 0.000000000000000000, -1.000000000000000000, 0.000000000000000000 ) ) ;
#4930=CARTESIAN_POINT ( 'NONE',  ( -17.18550143358999449, -2.500000000000000000, -495.8459145668000474 ) ) ;
#4940=ORIENTED_EDGE ( 'NONE', *, *, #27, .F. ) ;
#4946=CARTESIAN_POINT ( 'NONE',  ( -10.00000000000000000, -2.500000000000000000, -272.5000000000000000 ) ) ;
#4951=DIRECTION ( 'NONE',  ( 0.000000000000000000, 1.000000000000000000, 0.000000000000000000 ) ) ;
#4963=ORIENTED_EDGE ( 'NONE', *, *, #6072, .F. ) ;
#4965=ORIENTED_EDGE ( 'NONE', *, *, #1084, .T. ) ;
#4980=CARTESIAN_POINT ( 'NONE',  ( -16.98100918689000238, -2.633704000000000267, -439.4179428962999623 ) ) ;
#4982=AXIS2_PLACEMENT_3D ( 'NONE', #3823, #9280, #1047 ) ;
#4991=DIRECTION ( 'NONE',  ( -1.000000000000000000, 0.000000000000000000, 0.000000000000000000 ) ) ;
#5008=ORIENTED_EDGE ( 'NONE', *, *, #7600, .F. ) ;
#5009=ADVANCED_FACE ( 'NONE', ( #9359 ), #8690, .T. ) ;
#5015=ADVANCED_FACE ( 'NONE', ( #6888 ), #377, .F. ) ;
#5049=VERTEX_POINT ( 'NONE', #9559 ) ;
#5056=CARTESIAN_POINT ( 'NONE',  ( -26.82908671702000802, 2.500000000000000000, -441.1544246730000509 ) ) ;
#5076=ORIENTED_EDGE ( 'NONE', *, *, #6872, .T. ) ;
#5085=EDGE_CURVE ( 'NONE', #223, #4480, #10214, .T. ) ;
#5108=CARTESIAN_POINT ( 'NONE',  ( -28.01838671672000203, 2.500000000000000000, -497.7560445212000104 ) ) ;
#5121=VERTEX_POINT ( 'NONE', #7358 ) ;
#5141=EDGE_CURVE ( 'NONE', #6958, #223, #10372, .T. ) ;
#5165=CARTESIAN_POINT ( 'NONE',  ( -28.01838671672000203, -2.500000000000000000, -497.7560445212000104 ) ) ;
#5177=ORIENTED_EDGE ( 'NONE', *, *, #2590, .T. ) ;
#5183=DIRECTION ( 'NONE',  ( 1.000000000000000000, 0.000000000000000000, 0.000000000000000000 ) ) ;
#5190=LINE ( 'NONE', #3316, #5888 ) ;
#5195=LINE ( 'NONE', #7512, #4341 ) ;
#5218=VECTOR ( 'NONE', #4951, 1000.000000000000000 ) ;
#5233=EDGE_CURVE ( 'NONE', #5378, #4852, #1215, .T. ) ;
#5243=LINE ( 'NONE', #9437, #6689 ) ;
#5244=DIRECTION ( 'NONE',  ( 0.000000000000000000, -1.000000000000000000, 0.000000000000000000 ) ) ;
#5266=ADVANCED_FACE ( 'NONE', ( #2134 ), #4446, .T. ) ;
#5279=EDGE_CURVE ( 'NONE', #3553, #6229, #6960, .T. ) ;
#5282=LINE ( 'NONE', #8554, #2108 ) ;
#5303=DIRECTION ( 'NONE',  ( -1.000000000000000000, 0.000000000000000000, 0.000000000000000000 ) ) ;
#5328=ADVANCED_FACE ( 'NONE', ( #995 ), #5724, .F. ) ;
#5330=ORIENTED_EDGE ( 'NONE', *, *, #5085, .F. ) ;
#5339=VECTOR ( 'NONE', #305, 1000.000000000000000 ) ;
#5341=SURFACE_STYLE_USAGE ( .BOTH. , #7926 ) ;
#5368=EDGE_CURVE ( 'NONE', #8790, #9887, #7708, .T. ) ;
#5373=FACE_OUTER_BOUND ( 'NONE', #3387, .T. ) ;
#5376=CARTESIAN_POINT ( 'NONE',  ( -53.50011725782000127, 2.656480000000000175, -412.5186446566000313 ) ) ;
#5378=VERTEX_POINT ( 'NONE', #7121 ) ;
#5391=ORIENTED_EDGE ( 'NONE', *, *, #27, .T. ) ;
#5395=CARTESIAN_POINT ( 'NONE',  ( -17.01838671672000203, -2.500000000000000000, -497.7560445212000104 ) ) ;
#5398=( NAMED_UNIT ( * ) PLANE_ANGLE_UNIT ( ) SI_UNIT ( $, .RADIAN. ) );
#5436=CARTESIAN_POINT ( 'NONE',  ( -26.82908671702000802, 2.500000000000000000, -441.1544246730000509 ) ) ;
#5450=SURFACE_STYLE_FILL_AREA ( #7873 ) ;
#5477=AXIS2_PLACEMENT_3D ( 'NONE', #4980, #7454, #98 ) ;
#5478=CARTESIAN_POINT ( 'NONE',  ( -28.01838671672000203, 2.500000000000000000, -497.7560445212000104 ) ) ;
#5502=CIRCLE ( 'NONE', #878, 11.00000000000000000 ) ;
#5521=ORIENTED_EDGE ( 'NONE', *, *, #1752, .T. ) ;
#5529=DIRECTION ( 'NONE',  ( 0.000000000000000000, 1.000000000000000000, 0.000000000000000000 ) ) ;
#5535=CYLINDRICAL_SURFACE ( 'NONE', #6076, 10.00000000000000533 ) ;
#5545=ORIENTED_EDGE ( 'NONE', *, *, #6330, .F. ) ;
#5587=PRODUCT_CONTEXT ( 'NONE', #9006, 'mechanical' ) ;
#5590=DIRECTION ( 'NONE',  ( 0.000000000000000000, 0.000000000000000000, 1.000000000000000000 ) ) ;
#5592=CARTESIAN_POINT ( 'NONE',  ( 7.420201433257000545, 2.500000000000000000, -419.8948508258000061 ) ) ;
#5600=FACE_OUTER_BOUND ( 'NONE', #5945, .T. ) ;
#5601=UNCERTAINTY_MEASURE_WITH_UNIT (LENGTH_MEASURE( 1.000000000000000082E-05 ), #2217, 'distance_accuracy_value', 'NONE');
#5605=ADVANCED_FACE ( 'NONE', ( #3755 ), #378, .T. ) ;
#5607=ORIENTED_EDGE ( 'NONE', *, *, #1891, .F. ) ;
#5608=CARTESIAN_POINT ( 'NONE',  ( -50.24071243418999444, 2.500000000000000000, -414.3237589990000629 ) ) ;
#5620=CARTESIAN_POINT ( 'NONE',  ( -5.500000000000000000, -2.500000000000000000, -409.5000000000000568 ) ) ;
#5623=VECTOR ( 'NONE', #3025, 1000.000000000000000 ) ;
#5654=VERTEX_POINT ( 'NONE', #6225 ) ;
#5659=ORIENTED_EDGE ( 'NONE', *, *, #2872, .F. ) ;
#5688=EDGE_CURVE ( 'NONE', #9634, #2247, #10158, .T. ) ;
#5691=CARTESIAN_POINT ( 'NONE',  ( -14.00000000000000000, -2.500000000000000000, -380.4979246178999688 ) ) ;
#5694=PLANE ( 'NONE',  #8739 ) ;
#5724=CYLINDRICAL_SURFACE ( 'NONE', #87, 3.499999999999999556 ) ;
#5734=CARTESIAN_POINT ( 'NONE',  ( -43.24071243418999444, 2.500000000000000000, -414.3237589990000629 ) ) ;
#5757=CARTESIAN_POINT ( 'NONE',  ( -14.00000000000000000, -2.500000000000000000, -380.4979246178999688 ) ) ;
#5776=ORIENTED_EDGE ( 'NONE', *, *, #5233, .T. ) ;
#5780=FACE_OUTER_BOUND ( 'NONE', #1827, .T. ) ;
#5785=AXIS2_PLACEMENT_3D ( 'NONE', #8808, #10474, #4790 ) ;
#5811=VERTEX_POINT ( 'NONE', #6387 ) ;
#5814=CARTESIAN_POINT ( 'NONE',  ( -2.000000000000000000, 2.500000000000000000, -409.5000000000000568 ) ) ;
#5815=EDGE_LOOP ( 'NONE', ( #2285, #1437, #1903, #9448 ) ) ;
#5817=VECTOR ( 'NONE', #1736, 1000.000000000000000 ) ;
#5820=EDGE_CURVE ( 'NONE', #9461, #3582, #2944, .T. ) ;
#5855=DIRECTION ( 'NONE',  ( -0.3420201433256988555, 0.000000000000000000, 0.9396926207858975477 ) ) ;
#5866=ORIENTED_EDGE ( 'NONE', *, *, #10161, .F. ) ;
#5885=ADVANCED_FACE ( 'NONE', ( #8109 ), #5958, .F. ) ;
#5888=VECTOR ( 'NONE', #999, 1000.000000000000000 ) ;
#5891=FACE_OUTER_BOUND ( 'NONE', #34, .T. ) ;
#5916=DIRECTION ( 'NONE',  ( 0.000000000000000000, 0.000000000000000000, -1.000000000000000000 ) ) ;
#5924=VERTEX_POINT ( 'NONE', #9992 ) ;
#5932=EDGE_CURVE ( 'NONE', #6229, #3553, #9647, .T. ) ;
#5943=EDGE_CURVE ( 'NONE', #8573, #215, #6773, .T. ) ;
#5945=EDGE_LOOP ( 'NONE', ( #7614, #8450, #6249, #10027 ) ) ;
#5952=CARTESIAN_POINT ( 'NONE',  ( -10.00000000000000000, -2.500000000000000000, -272.5000000000000000 ) ) ;
#5958=CYLINDRICAL_SURFACE ( 'NONE', #4492, 3.500000000000003109 ) ;
#5992=ORIENTED_EDGE ( 'NONE', *, *, #5820, .T. ) ;
#6010=CIRCLE ( 'NONE', #3442, 3.500000000000003109 ) ;
#6013=CIRCLE ( 'NONE', #6533, 10.00000000000000000 ) ;
#6070=AXIS2_PLACEMENT_3D ( 'NONE', #3749, #9720, #10310 ) ;
#6071=CARTESIAN_POINT ( 'NONE',  ( -38.59226537204000351, -2.500000000000000000, -500.7880554352000217 ) ) ;
#6072=EDGE_CURVE ( 'NONE', #2769, #5378, #9483, .T. ) ;
#6076=AXIS2_PLACEMENT_3D ( 'NONE', #5376, #8818, #3826 ) ;
#6078=VECTOR ( 'NONE', #6119, 1000.000000000000000 ) ;
#6093=CARTESIAN_POINT ( 'NONE',  ( -20.57979856674000629, -2.500000000000000000, -389.8948508258000061 ) ) ;
#6119=DIRECTION ( 'NONE',  ( 0.000000000000000000, 1.000000000000000000, 0.000000000000000000 ) ) ;
#6126=LINE ( 'NONE', #10162, #4263 ) ;
#6146=VERTEX_POINT ( 'NONE', #4002 ) ;
#6164=CARTESIAN_POINT ( 'NONE',  ( -43.24071243418999444, 2.500000000000000000, -414.3237589990000629 ) ) ;
#6198=ORIENTED_EDGE ( 'NONE', *, *, #757, .T. ) ;
#6225=CARTESIAN_POINT ( 'NONE',  ( 1.499999999999999556, 2.500000000000000000, -409.5000000000000568 ) ) ;
#6229=VERTEX_POINT ( 'NONE', #5608 ) ;
#6244=CIRCLE ( 'NONE', #3672, 10.00000000000000533 ) ;
#6248=AXIS2_PLACEMENT_3D ( 'NONE', #3231, #9678, #658 ) ;
#6249=ORIENTED_EDGE ( 'NONE', *, *, #2872, .T. ) ;
#6251=PLANE ( 'NONE',  #9357 ) ;
#6253=EDGE_CURVE ( 'NONE', #6326, #5811, #1529, .T. ) ;
#6254=ORIENTED_EDGE ( 'NONE', *, *, #2542, .F. ) ;
#6262=SHAPE_REPRESENTATION_RELATIONSHIP ( 'NONE' , 'NONE' ,  #6273, #3778 ) ;
#6273=SHAPE_REPRESENTATION ( 'Lower Jaw Base Arm', ( #2817 ), #7476 ) ;
#6275=PLANE ( 'NONE',  #1684 ) ;
#6278=PRODUCT_DEFINITION_FORMATION_WITH_SPECIFIED_SOURCE ( 'ANY', '', #1924, .NOT_KNOWN. ) ;
#6287=VECTOR ( 'NONE', #5916, 1000.000000000000000 ) ;
#6298=FACE_BOUND ( 'NONE', #502, .T. ) ;
#6325=CARTESIAN_POINT ( 'NONE',  ( -37.87192209818999800, 2.500000000000000000, -461.0868123482000556 ) ) ;
#6326=VERTEX_POINT ( 'NONE', #9912 ) ;
#6330=EDGE_CURVE ( 'NONE', #6416, #5654, #555, .T. ) ;
#6334=LINE ( 'NONE', #5691, #1510 ) ;
#6335=CIRCLE ( 'NONE', #1194, 3.500000000000003109 ) ;
#6336=VECTOR ( 'NONE', #678, 1000.000000000000000 ) ;
#6353=ORIENTED_EDGE ( 'NONE', *, *, #9179, .T. ) ;
#6355=AXIS2_PLACEMENT_3D ( 'NONE', #7190, #3100, #742 ) ;
#6357=EDGE_LOOP ( 'NONE', ( #7542, #4495, #7074, #8734 ) ) ;
#6362=ORIENTED_EDGE ( 'NONE', *, *, #3844, .F. ) ;
#6387=CARTESIAN_POINT ( 'NONE',  ( -14.00000000000000000, 2.500000000000000000, -317.5000000000000000 ) ) ;
#6392=VECTOR ( 'NONE', #3639, 1000.000000000000227 ) ;
#6401=DIRECTION ( 'NONE',  ( 0.000000000000000000, -1.000000000000000000, 0.000000000000000000 ) ) ;
#6403=( NAMED_UNIT ( * ) SI_UNIT ( $, .STERADIAN. ) SOLID_ANGLE_UNIT ( ) );
#6408=VECTOR ( 'NONE', #41, 1000.000000000000000 ) ;
#6413=DIRECTION ( 'NONE',  ( 1.000000000000000000, 0.000000000000000000, 0.000000000000000000 ) ) ;
#6416=VERTEX_POINT ( 'NONE', #4376 ) ;
#6420=AXIS2_PLACEMENT_3D ( 'NONE', #2447, #831, #4110 ) ;
#6427=ORIENTED_EDGE ( 'NONE', *, *, #1807, .T. ) ;
#6443=VERTEX_POINT ( 'NONE', #244 ) ;
#6467=EDGE_LOOP ( 'NONE', ( #3197, #5545, #4120, #6537 ) ) ;
#6468=LINE ( 'NONE', #3999, #10184 ) ;
#6476=ADVANCED_FACE ( 'NONE', ( #7649 ), #3518, .T. ) ;
#6501=DIRECTION ( 'NONE',  ( 0.000000000000000000, 1.000000000000000000, 0.000000000000000000 ) ) ;
#6506=SHAPE_DEFINITION_REPRESENTATION ( #4412, #6273 ) ;
#6529=CARTESIAN_POINT ( 'NONE',  ( 10.00000000000000000, -2.500000000000000000, -317.5000000000000000 ) ) ;
#6533=AXIS2_PLACEMENT_3D ( 'NONE', #9469, #1245, #610 ) ;
#6537=ORIENTED_EDGE ( 'NONE', *, *, #7705, .T. ) ;
#6544=CARTESIAN_POINT ( 'NONE',  ( -30.87192209819000155, 2.500000000000000000, -461.0868123482000556 ) ) ;
#6552=CARTESIAN_POINT ( 'NONE',  ( -38.59226537204000351, 2.500000000000000000, -500.7880554352000217 ) ) ;
#6569=CARTESIAN_POINT ( 'NONE',  ( 7.420201433257000545, -2.500000000000000000, -419.8948508258000061 ) ) ;
#6576=VERTEX_POINT ( 'NONE', #9375 ) ;
#6590=DIRECTION ( 'NONE',  ( 1.000000000000000000, 0.000000000000000000, 0.000000000000000000 ) ) ;
#6614=EDGE_CURVE ( 'NONE', #7746, #9766, #7699, .T. ) ;
#6644=DIRECTION ( 'NONE',  ( 1.000000000000000000, 0.000000000000000000, 0.000000000000000000 ) ) ;
#6662=ORIENTED_EDGE ( 'NONE', *, *, #8571, .T. ) ;
#6665=LINE ( 'NONE', #4354, #4772 ) ;
#6674=CARTESIAN_POINT ( 'NONE',  ( -24.00000000000000000, 2.500000000000000000, -380.4979246178999688 ) ) ;
#6677=EDGE_CURVE ( 'NONE', #6416, #9387, #4522, .T. ) ;
#6689=VECTOR ( 'NONE', #4484, 1000.000000000000000 ) ;
#6696=ORIENTED_EDGE ( 'NONE', *, *, #6614, .F. ) ;
#6714=ORIENTED_EDGE ( 'NONE', *, *, #1595, .T. ) ;
#6733=DIRECTION ( 'NONE',  ( 0.000000000000000000, 1.000000000000000000, 0.000000000000000000 ) ) ;
#6734=EDGE_CURVE ( 'NONE', #3477, #1984, #2419, .T. ) ;
#6757=CARTESIAN_POINT ( 'NONE',  ( -46.74071243419000155, 2.500000000000000000, -414.3237589990000629 ) ) ;
#6766=( NAMED_UNIT ( * ) PLANE_ANGLE_UNIT ( ) SI_UNIT ( $, .RADIAN. ) );
#6767=DIRECTION ( 'NONE',  ( 1.000000000000000000, 0.000000000000000000, 0.000000000000000000 ) ) ;
#6773=LINE ( 'NONE', #8425, #8436 ) ;
#6776=CLOSED_SHELL ( 'NONE', ( #1239, #5266, #7292, #9838, #7012, #5605, #1667, #4122, #3803, #8696, #2828, #10609, #8704, #7806, #2504, #6476, #5009, #2120, #3397, #1801, #5328, #2246, #5015, #2078, #3204, #5885, #1277 ) ) ;
#6790=CYLINDRICAL_SURFACE ( 'NONE', #4064, 11.00000000000000000 ) ;
#6795=EDGE_LOOP ( 'NONE', ( #6714, #4218 ) ) ;
#6798=ORIENTED_EDGE ( 'NONE', *, *, #4052, .T. ) ;
#6799=DIRECTION ( 'NONE',  ( 1.000000000000000000, 0.000000000000000000, 0.000000000000000000 ) ) ;
#6814=EDGE_CURVE ( 'NONE', #886, #7746, #6010, .T. ) ;
#6820=DIRECTION ( 'NONE',  ( 1.000000000000000000, 0.000000000000000000, 0.000000000000000000 ) ) ;
#6829=DIRECTION ( 'NONE',  ( 0.000000000000000000, 0.000000000000000000, -1.000000000000000000 ) ) ;
#6842=CYLINDRICAL_SURFACE ( 'NONE', #1324, 3.500000000000003109 ) ;
#6849=EDGE_CURVE ( 'NONE', #4552, #4872, #7050, .T. ) ;
#6864=EDGE_LOOP ( 'NONE', ( #7281, #9780, #7756, #2636 ) ) ;
#6872=EDGE_CURVE ( 'NONE', #5811, #5378, #580, .T. ) ;
#6888=FACE_OUTER_BOUND ( 'NONE', #877, .T. ) ;
#6893=CARTESIAN_POINT ( 'NONE',  ( 14.00000000000000000, -2.500000000000000000, -272.5000000000000000 ) ) ;
#6902=DIRECTION ( 'NONE',  ( 0.000000000000000000, -1.000000000000000000, 0.000000000000000000 ) ) ;
#6931=EDGE_CURVE ( 'NONE', #8108, #10456, #9264, .T. ) ;
#6943=FACE_OUTER_BOUND ( 'NONE', #4471, .T. ) ;
#6948=DIRECTION ( 'NONE',  ( 0.000000000000000000, -1.000000000000000000, 0.000000000000000000 ) ) ;
#6958=VERTEX_POINT ( 'NONE', #4930 ) ;
#6960=CIRCLE ( 'NONE', #940, 3.500000000000003109 ) ;
#6962=FACE_BOUND ( 'NONE', #110, .T. ) ;
#6971=CARTESIAN_POINT ( 'NONE',  ( 1.499999999999999556, -2.500000000000000000, -409.5000000000000568 ) ) ;
#6992=CARTESIAN_POINT ( 'NONE',  ( -20.40121062015000319, -2.500000000000000000, -430.0210166885000262 ) ) ;
#7006=DIRECTION ( 'NONE',  ( 0.000000000000000000, 0.000000000000000000, -1.000000000000000000 ) ) ;
#7007=DIRECTION ( 'NONE',  ( 1.000000000000000000, 0.000000000000000000, 0.000000000000000000 ) ) ;
#7012=ADVANCED_FACE ( 'NONE', ( #1496 ), #2358, .T. ) ;
#7016=VERTEX_POINT ( 'NONE', #6544 ) ;
#7036=DIRECTION ( 'NONE',  ( 0.000000000000000000, -1.000000000000000000, 0.000000000000000000 ) ) ;
#7040=CYLINDRICAL_SURFACE ( 'NONE', #2958, 3.500000000000003109 ) ;
#7050=CIRCLE ( 'NONE', #8753, 3.500000000000003109 ) ;
#7067=PLANE ( 'NONE',  #8697 ) ;
#7072=ORIENTED_EDGE ( 'NONE', *, *, #5368, .T. ) ;
#7074=ORIENTED_EDGE ( 'NONE', *, *, #5368, .F. ) ;
#7095=DIRECTION ( 'NONE',  ( -1.000000000000000000, 0.000000000000000000, 0.000000000000000000 ) ) ;
#7098=DIRECTION ( 'NONE',  ( 0.000000000000000000, -1.000000000000000000, 0.000000000000000000 ) ) ;
#7121=CARTESIAN_POINT ( 'NONE',  ( -10.00000000000000000, 2.500000000000000000, -317.5000000000000000 ) ) ;
#7129=EDGE_CURVE ( 'NONE', #10404, #9387, #360, .T. ) ;
#7184=ORIENTED_EDGE ( 'NONE', *, *, #5688, .T. ) ;
#7187=ORIENTED_EDGE ( 'NONE', *, *, #5943, .F. ) ;
#7190=CARTESIAN_POINT ( 'NONE',  ( -28.01838671672000203, -2.500000000000000000, -497.7560445212000104 ) ) ;
#7221=ORIENTED_EDGE ( 'NONE', *, *, #4052, .F. ) ;
#7279=ORIENTED_EDGE ( 'NONE', *, *, #114, .T. ) ;
#7281=ORIENTED_EDGE ( 'NONE', *, *, #7776, .T. ) ;
#7283=VERTEX_POINT ( 'NONE', #2516 ) ;
#7289=CARTESIAN_POINT ( 'NONE',  ( -50.24071243418999444, -2.500000000000000000, -414.3237589990000629 ) ) ;
#7292=ADVANCED_FACE ( 'NONE', ( #5780 ), #1707, .F. ) ;
#7350=VECTOR ( 'NONE', #440, 1000.000000000000000 ) ;
#7358=CARTESIAN_POINT ( 'NONE',  ( -20.40121062015000319, -2.500000000000000000, -430.0210166885000262 ) ) ;
#7370=CARTESIAN_POINT ( 'NONE',  ( 10.00000000000000000, -2.500000000000000000, -272.5000000000000000 ) ) ;
#7394=AXIS2_PLACEMENT_3D ( 'NONE', #10573, #1654, #4129 ) ;
#7395=VECTOR ( 'NONE', #8987, 1000.000000000000000 ) ;
#7413=DIRECTION ( 'NONE',  ( 0.000000000000000000, -1.000000000000000000, 0.000000000000000000 ) ) ;
#7414=ORIENTED_EDGE ( 'NONE', *, *, #6677, .F. ) ;
#7422=DIRECTION ( 'NONE',  ( 0.000000000000000000, -1.000000000000000000, 0.000000000000000000 ) ) ;
#7454=DIRECTION ( 'NONE',  ( 0.000000000000000000, 1.000000000000000000, 0.000000000000000000 ) ) ;
#7467=ORIENTED_EDGE ( 'NONE', *, *, #6253, .T. ) ;
#7476=( GEOMETRIC_REPRESENTATION_CONTEXT ( 3 ) GLOBAL_UNCERTAINTY_ASSIGNED_CONTEXT ( ( #2705 ) ) GLOBAL_UNIT_ASSIGNED_CONTEXT ( ( #4488, #6766, #7671 ) ) REPRESENTATION_CONTEXT ( 'NONE', 'WORKASPACE' ) );
#7494=ORIENTED_EDGE ( 'NONE', *, *, #8843, .F. ) ;
#7512=CARTESIAN_POINT ( 'NONE',  ( 10.00000000000000000, -2.500000000000000000, -317.5000000000000000 ) ) ;
#7517=DIRECTION ( 'NONE',  ( 0.000000000000000000, -1.000000000000000000, 0.000000000000000000 ) ) ;
#7519=VERTEX_POINT ( 'NONE', #9747 ) ;
#7534=DIRECTION ( 'NONE',  ( -1.000000000000000000, 0.000000000000000000, 0.000000000000000000 ) ) ;
#7542=ORIENTED_EDGE ( 'NONE', *, *, #507, .T. ) ;
#7573=DIRECTION ( 'NONE',  ( 0.000000000000000000, 1.000000000000000000, 0.000000000000000000 ) ) ;
#7588=AXIS2_PLACEMENT_3D ( 'NONE', #5814, #9807, #931 ) ;
#7600=EDGE_CURVE ( 'NONE', #8108, #215, #2706, .T. ) ;
#7601=VECTOR ( 'NONE', #1474, 1000.000000000000000 ) ;
#7614=ORIENTED_EDGE ( 'NONE', *, *, #2317, .F. ) ;
#7626=AXIS2_PLACEMENT_3D ( 'NONE', #10263, #8583, #9408 ) ;
#7631=ORIENTED_EDGE ( 'NONE', *, *, #4776, .T. ) ;
#7649=FACE_OUTER_BOUND ( 'NONE', #1647, .T. ) ;
#7658=DIRECTION ( 'NONE',  ( 0.000000000000000000, -1.000000000000000000, 0.000000000000000000 ) ) ;
#7665=ORIENTED_EDGE ( 'NONE', *, *, #9880, .T. ) ;
#7671=( NAMED_UNIT ( * ) SI_UNIT ( $, .STERADIAN. ) SOLID_ANGLE_UNIT ( ) );
#7699=LINE ( 'NONE', #2916, #731 ) ;
#7705=EDGE_CURVE ( 'NONE', #9387, #10404, #4290, .T. ) ;
#7706=CARTESIAN_POINT ( 'NONE',  ( -34.37192209818999800, 2.500000000000000000, -461.0868123482000556 ) ) ;
#7708=LINE ( 'NONE', #1049, #7803 ) ;
#7735=DIRECTION ( 'NONE',  ( -1.000000000000000000, 0.000000000000000000, 0.000000000000000000 ) ) ;
#7746=VERTEX_POINT ( 'NONE', #8442 ) ;
#7754=DIRECTION ( 'NONE',  ( 0.000000000000000000, 1.000000000000000000, 0.000000000000000000 ) ) ;
#7756=ORIENTED_EDGE ( 'NONE', *, *, #507, .F. ) ;
#7759=ORIENTED_EDGE ( 'NONE', *, *, #5820, .F. ) ;
#7761=ORIENTED_EDGE ( 'NONE', *, *, #5279, .T. ) ;
#7775=CARTESIAN_POINT ( 'NONE',  ( -53.50011725782000127, 2.500000000000000000, -412.5186446566000313 ) ) ;
#7776=EDGE_CURVE ( 'NONE', #4332, #289, #338, .T. ) ;
#7791=VECTOR ( 'NONE', #3870, 1000.000000000000000 ) ;
#7803=VECTOR ( 'NONE', #10181, 1000.000000000000000 ) ;
#7806=ADVANCED_FACE ( 'NONE', ( #657 ), #5694, .T. ) ;
#7824=ORIENTED_EDGE ( 'NONE', *, *, #7776, .F. ) ;
#7844=AXIS2_PLACEMENT_3D ( 'NONE', #8010, #10529, #3174 ) ;
#7845=ORIENTED_EDGE ( 'NONE', *, *, #8827, .F. ) ;
#7860=DIRECTION ( 'NONE',  ( -0.000000000000000000, 1.000000000000000000, 0.000000000000000000 ) ) ;
#7873=FILL_AREA_STYLE ('',( #522 ) ) ;
#7884=ORIENTED_EDGE ( 'NONE', *, *, #10174, .T. ) ;
#7898=CARTESIAN_POINT ( 'NONE',  ( -28.01838671672000203, 2.500000000000000000, -497.7560445212000104 ) ) ;
#7910=LINE ( 'NONE', #4474, #5623 ) ;
#7926=SURFACE_SIDE_STYLE ('',( #5450 ) ) ;
#7938=CARTESIAN_POINT ( 'NONE',  ( -14.00000000000000000, 2.500000000000000000, -317.5000000000000000 ) ) ;
#7944=CARTESIAN_POINT ( 'NONE',  ( -46.74071243419000155, 2.500000000000000000, -414.3237589990000629 ) ) ;
#7961=CARTESIAN_POINT ( 'NONE',  ( -14.00000000000000000, -2.500000000000000000, -387.5000000000000000 ) ) ;
#7963=CARTESIAN_POINT ( 'NONE',  ( -2.000000000000000000, 2.500000000000000000, -409.5000000000000568 ) ) ;
#7964=AXIS2_PLACEMENT_3D ( 'NONE', #10268, #2905, #4569 ) ;
#7970=VECTOR ( 'NONE', #1027, 1000.000000000000000 ) ;
#7972=FACE_BOUND ( 'NONE', #6795, .T. ) ;
#7974=VECTOR ( 'NONE', #7006, 1000.000000000000000 ) ;
#7982=ORIENTED_EDGE ( 'NONE', *, *, #5932, .F. ) ;
#7988=PRESENTATION_STYLE_ASSIGNMENT (( #5341 ) ) ;
#8004=CARTESIAN_POINT ( 'NONE',  ( -28.01838671672000203, -2.500000000000000000, -497.7560445212000104 ) ) ;
#8007=CARTESIAN_POINT ( 'NONE',  ( -24.00000000000000000, -2.500000000000000000, -380.4979246178999688 ) ) ;
#8010=CARTESIAN_POINT ( 'NONE',  ( -46.74071243419000155, -2.500000000000000000, -414.3237589990000629 ) ) ;
#8033=LINE ( 'NONE', #6529, #6336 ) ;
#8037=ORIENTED_EDGE ( 'NONE', *, *, #5688, .F. ) ;
#8061=VECTOR ( 'NONE', #8300, 1000.000000000000000 ) ;
#8069=FACE_OUTER_BOUND ( 'NONE', #2526, .T. ) ;
#8087=CARTESIAN_POINT ( 'NONE',  ( -17.01838671672000203, 2.500000000000000000, -497.7560445212000104 ) ) ;
#8100=AXIS2_PLACEMENT_3D ( 'NONE', #1143, #6799, #2111 ) ;
#8108=VERTEX_POINT ( 'NONE', #376 ) ;
#8109=FACE_OUTER_BOUND ( 'NONE', #2389, .T. ) ;
#8121=CARTESIAN_POINT ( 'NONE',  ( -34.37192209818999800, 2.500000000000000000, -461.0868123482000556 ) ) ;
#8176=CARTESIAN_POINT ( 'NONE',  ( -30.87192209819000155, -2.500000000000000000, -461.0868123482000556 ) ) ;
#8199=EDGE_LOOP ( 'NONE', ( #2774, #3027 ) ) ;
#8217=DIRECTION ( 'NONE',  ( -0.9396926207858972147, 0.000000000000000000, -0.3420201433256990775 ) ) ;
#8223=CARTESIAN_POINT ( 'NONE',  ( -10.00000000000000000, -2.500000000000000000, -272.5000000000000000 ) ) ;
#8225=DIRECTION ( 'NONE',  ( -1.000000000000000000, 0.000000000000000000, 0.000000000000000000 ) ) ;
#8227=ORIENTED_EDGE ( 'NONE', *, *, #5943, .T. ) ;
#8229=PRODUCT_DEFINITION ( 'UNKNOWN', '', #6278, #2600 ) ;
#8236=CIRCLE ( 'NONE', #4982, 10.00000000000000000 ) ;
#8240=ORIENTED_EDGE ( 'NONE', *, *, #3455, .F. ) ;
#8271=DIRECTION ( 'NONE',  ( 1.000000000000000000, 0.000000000000000000, 0.000000000000000000 ) ) ;
#8300=DIRECTION ( 'NONE',  ( -1.705302565823999938E-14, -1.000000000000000000, -0.000000000000000000 ) ) ;
#8309=CIRCLE ( 'NONE', #6420, 10.00000000000000533 ) ;
#8312=CIRCLE ( 'NONE', #3670, 3.500000000000003109 ) ;
#8318=DIRECTION ( 'NONE',  ( 0.000000000000000000, 1.000000000000000000, 0.000000000000000000 ) ) ;
#8370=VECTOR ( 'NONE', #8217, 1000.000000000000227 ) ;
#8390=FACE_BOUND ( 'NONE', #8199, .T. ) ;
#8391=FACE_OUTER_BOUND ( 'NONE', #5815, .T. ) ;
#8395=ORIENTED_EDGE ( 'NONE', *, *, #8443, .T. ) ;
#8409=ORIENTED_EDGE ( 'NONE', *, *, #6614, .T. ) ;
#8425=CARTESIAN_POINT ( 'NONE',  ( -38.59226537204000351, -2.500000000000000000, -500.7880554352000217 ) ) ;
#8427=LINE ( 'NONE', #3550, #816 ) ;
#8436=VECTOR ( 'NONE', #1065, 1000.000000000000000 ) ;
#8438=LINE ( 'NONE', #4365, #6287 ) ;
#8442=CARTESIAN_POINT ( 'NONE',  ( -24.51838671671999847, 2.500000000000000000, -497.7560445212000104 ) ) ;
#8443=EDGE_CURVE ( 'NONE', #10456, #6576, #885, .T. ) ;
#8450=ORIENTED_EDGE ( 'NONE', *, *, #5279, .F. ) ;
#8477=EDGE_LOOP ( 'NONE', ( #6198, #2551, #2819, #2633 ) ) ;
#8479=CIRCLE ( 'NONE', #10205, 3.499999999999999556 ) ;
#8494=EDGE_CURVE ( 'NONE', #344, #4674, #6335, .T. ) ;
#8523=DIRECTION ( 'NONE',  ( 0.000000000000000000, 0.000000000000000000, 1.000000000000000000 ) ) ;
#8550=ORIENTED_EDGE ( 'NONE', *, *, #2556, .F. ) ;
#8553=DIRECTION ( 'NONE',  ( 0.9848077530122130163, 0.000000000000000000, 0.1736481776669023813 ) ) ;
#8554=CARTESIAN_POINT ( 'NONE',  ( -17.18550143358999449, -2.500000000000000000, -495.8459145668000474 ) ) ;
#8571=EDGE_CURVE ( 'NONE', #6443, #5121, #8236, .T. ) ;
#8573=VERTEX_POINT ( 'NONE', #10127 ) ;
#8583=DIRECTION ( 'NONE',  ( 0.000000000000000000, -1.000000000000000000, 0.000000000000000000 ) ) ;
#8585=DIRECTION ( 'NONE',  ( 0.000000000000000000, 1.000000000000000000, 0.000000000000000000 ) ) ;
#8596=FILL_AREA_STYLE_COLOUR ( '', #1381 ) ;
#8599=ORIENTED_EDGE ( 'NONE', *, *, #4128, .F. ) ;
#8612=EDGE_LOOP ( 'NONE', ( #2993, #715 ) ) ;
#8632=VERTEX_POINT ( 'NONE', #2162 ) ;
#8634=CARTESIAN_POINT ( 'NONE',  ( 0.000000000000000000, 0.000000000000000000, 0.000000000000000000 ) ) ;
#8644=LINE ( 'NONE', #1290, #3848 ) ;
#8648=AXIS2_PLACEMENT_3D ( 'NONE', #1285, #7098, #9508 ) ;
#8658=ORIENTED_EDGE ( 'NONE', *, *, #1891, .T. ) ;
#8659=VECTOR ( 'NONE', #8523, 1000.000000000000000 ) ;
#8663=EDGE_LOOP ( 'NONE', ( #1273, #9029, #8658, #8037 ) ) ;
#8690=CYLINDRICAL_SURFACE ( 'NONE', #8648, 10.00000000000000533 ) ;
#8696=ADVANCED_FACE ( 'NONE', ( #5373 ), #4686, .T. ) ;
#8697=AXIS2_PLACEMENT_3D ( 'NONE', #9476, #7860, #506 ) ;
#8704=ADVANCED_FACE ( 'NONE', ( #608 ), #3180, .T. ) ;
#8705=DIRECTION ( 'NONE',  ( -1.000000000000000000, 0.000000000000000000, 0.000000000000000000 ) ) ;
#8718=DIRECTION ( 'NONE',  ( 0.000000000000000000, -1.000000000000000000, 0.000000000000000000 ) ) ;
#8725=CARTESIAN_POINT ( 'NONE',  ( -63.11273421720001409, -2.500000000000000000, -415.2750182148000135 ) ) ;
#8734=ORIENTED_EDGE ( 'NONE', *, *, #1223, .T. ) ;
#8739=AXIS2_PLACEMENT_3D ( 'NONE', #3931, #8871, #8813 ) ;
#8742=CARTESIAN_POINT ( 'NONE',  ( -38.59226537204000351, -2.500000000000000000, -500.7880554352000217 ) ) ;
#8753=AXIS2_PLACEMENT_3D ( 'NONE', #3506, #7036, #5303 ) ;
#8766=VERTEX_POINT ( 'NONE', #1673 ) ;
#8773=VERTEX_POINT ( 'NONE', #4946 ) ;
#8790=VERTEX_POINT ( 'NONE', #7370 ) ;
#8794=EDGE_LOOP ( 'NONE', ( #7072, #10270, #1447, #5177 ) ) ;
#8802=DIRECTION ( 'NONE',  ( 0.000000000000000000, 1.000000000000000000, 0.000000000000000000 ) ) ;
#8808=CARTESIAN_POINT ( 'NONE',  ( 10.00000000000000000, -2.500000000000000000, -317.5000000000000000 ) ) ;
#8813=DIRECTION ( 'NONE',  ( 0.000000000000000000, 0.000000000000000000, -1.000000000000000000 ) ) ;
#8818=DIRECTION ( 'NONE',  ( 0.000000000000000000, -1.000000000000000000, 0.000000000000000000 ) ) ;
#8827=EDGE_CURVE ( 'NONE', #9158, #7016, #8312, .T. ) ;
#8829=DIRECTION ( 'NONE',  ( -1.000000000000000000, 0.000000000000000000, 0.000000000000000000 ) ) ;
#8843=EDGE_CURVE ( 'NONE', #4872, #4552, #8479, .T. ) ;
#8868=ORIENTED_EDGE ( 'NONE', *, *, #3844, .T. ) ;
#8871=DIRECTION ( 'NONE',  ( 1.000000000000000000, 0.000000000000000000, 0.000000000000000000 ) ) ;
#8881=CARTESIAN_POINT ( 'NONE',  ( -46.74071243419000155, 2.500000000000000000, -414.3237589990000629 ) ) ;
#8940=ORIENTED_EDGE ( 'NONE', *, *, #5141, .T. ) ;
#8979=DIRECTION ( 'NONE',  ( 0.000000000000000000, 1.000000000000000000, 0.000000000000000000 ) ) ;
#8984=CARTESIAN_POINT ( 'NONE',  ( -34.37192209818999800, -2.500000000000000000, -461.0868123482000556 ) ) ;
#8987=DIRECTION ( 'NONE',  ( 0.1736481776669025201, 0.000000000000000000, -0.9848077530122130163 ) ) ;
#8991=LINE ( 'NONE', #5757, #1539 ) ;
#9002=EDGE_LOOP ( 'NONE', ( #7494, #1479 ) ) ;
#9006=APPLICATION_CONTEXT ( 'automotive_design' ) ;
#9015=ORIENTED_EDGE ( 'NONE', *, *, #6253, .F. ) ;
#9028=DIRECTION ( 'NONE',  ( 0.3420201433256988555, 0.000000000000000000, -0.9396926207858975477 ) ) ;
#9029=ORIENTED_EDGE ( 'NONE', *, *, #1752, .F. ) ;
#9040=EDGE_CURVE ( 'NONE', #6576, #3582, #537, .T. ) ;
#9042=LINE ( 'NONE', #177, #5218 ) ;
#9047=EDGE_CURVE ( 'NONE', #7746, #886, #1621, .T. ) ;
#9062=EDGE_CURVE ( 'NONE', #5121, #3477, #1229, .T. ) ;
#9092=VECTOR ( 'NONE', #9850, 1000.000000000000227 ) ;
#9106=AXIS2_PLACEMENT_3D ( 'NONE', #8223, #5590, #7422 ) ;
#9118=ORIENTED_EDGE ( 'NONE', *, *, #113, .T. ) ;
#9127=VECTOR ( 'NONE', #4898, 1000.000000000000000 ) ;
#9134=EDGE_LOOP ( 'NONE', ( #9991, #4536 ) ) ;
#9146=AXIS2_PLACEMENT_3D ( 'NONE', #7706, #7658, #5183 ) ;
#9158=VERTEX_POINT ( 'NONE', #6325 ) ;
#9177=CARTESIAN_POINT ( 'NONE',  ( -31.51838671672000558, 2.500000000000000000, -497.7560445212000104 ) ) ;
#9179=EDGE_CURVE ( 'NONE', #5049, #8108, #2418, .T. ) ;
#9184=ORIENTED_EDGE ( 'NONE', *, *, #1223, .F. ) ;
#9193=CARTESIAN_POINT ( 'NONE',  ( -46.74071243419000155, 2.500000000000000000, -414.3237589990000629 ) ) ;
#9198=CARTESIAN_POINT ( 'NONE',  ( -28.01838671672000203, 2.500000000000000000, -497.7560445212000104 ) ) ;
#9209=DIRECTION ( 'NONE',  ( 1.000000000000000000, 0.000000000000000000, 0.000000000000000000 ) ) ;
#9230=CARTESIAN_POINT ( 'NONE',  ( -2.000000000000000000, 2.500000000000000000, -409.5000000000000568 ) ) ;
#9243=AXIS2_PLACEMENT_3D ( 'NONE', #7898, #5529, #1185 ) ;
#9249=EDGE_LOOP ( 'NONE', ( #10522, #7631, #6362, #8395 ) ) ;
#9264=CIRCLE ( 'NONE', #187, 10.00000000000000000 ) ;
#9280=DIRECTION ( 'NONE',  ( 0.000000000000000000, 1.000000000000000000, 0.000000000000000000 ) ) ;
#9284=EDGE_LOOP ( 'NONE', ( #2576, #10497, #10286, #2512 ) ) ;
#9290=( GEOMETRIC_REPRESENTATION_CONTEXT ( 3 ) GLOBAL_UNCERTAINTY_ASSIGNED_CONTEXT ( ( #5601 ) ) GLOBAL_UNIT_ASSIGNED_CONTEXT ( ( #2217, #10483, #6403 ) ) REPRESENTATION_CONTEXT ( 'NONE', 'WORKASPACE' ) );
#9296=CARTESIAN_POINT ( 'NONE',  ( 14.00000000000000000, -2.500000000000000000, -317.5000000000000000 ) ) ;
#9312=AXIS2_PLACEMENT_3D ( 'NONE', #6071, #10217, #8585 ) ;
#9318=AXIS2_PLACEMENT_3D ( 'NONE', #5478, #3820, #3012 ) ;
#9319=ORIENTED_EDGE ( 'NONE', *, *, #1940, .F. ) ;
#9343=CARTESIAN_POINT ( 'NONE',  ( -56.92031869107000119, 2.500000000000000000, -403.1217184488000385 ) ) ;
#9347=EDGE_LOOP ( 'NONE', ( #5330, #3623, #2814, #2977 ) ) ;
#9348=AXIS2_PLACEMENT_3D ( 'NONE', #7963, #1465, #7007 ) ;
#9357=AXIS2_PLACEMENT_3D ( 'NONE', #2174, #723, #8718 ) ;
#9359=FACE_OUTER_BOUND ( 'NONE', #8663, .T. ) ;
#9365=FACE_BOUND ( 'NONE', #8612, .T. ) ;
#9367=( GEOMETRIC_REPRESENTATION_CONTEXT ( 3 ) GLOBAL_UNCERTAINTY_ASSIGNED_CONTEXT ( ( #17 ) ) GLOBAL_UNIT_ASSIGNED_CONTEXT ( ( #9490, #5398, #10448 ) ) REPRESENTATION_CONTEXT ( 'NONE', 'WORKASPACE' ) );
#9375=CARTESIAN_POINT ( 'NONE',  ( -56.92031869107000119, -2.500000000000000000, -403.1217184488000385 ) ) ;
#9387=VERTEX_POINT ( 'NONE', #5620 ) ;
#9397=EDGE_LOOP ( 'NONE', ( #4058, #403, #7279, #10067, #4642, #6353, #4523, #8868, #9118, #7467, #5076, #5776, #7665, #9994, #2984, #3785, #5521 ) ) ;
#9401=DIRECTION ( 'NONE',  ( 1.000000000000000000, 0.000000000000000000, 0.000000000000000000 ) ) ;
#9408=DIRECTION ( 'NONE',  ( 1.000000000000000000, 0.000000000000000000, 0.000000000000000000 ) ) ;
#9437=CARTESIAN_POINT ( 'NONE',  ( -14.00000000000000000, -2.500000000000000000, -317.5000000000000000 ) ) ;
#9440=AXIS2_PLACEMENT_3D ( 'NONE', #7961, #8705, #4631 ) ;
#9448=ORIENTED_EDGE ( 'NONE', *, *, #8843, .T. ) ;
#9461=VERTEX_POINT ( 'NONE', #9765 ) ;
#9467=AXIS2_PLACEMENT_3D ( 'NONE', #853, #2472, #9028 ) ;
#9469=CARTESIAN_POINT ( 'NONE',  ( 4.000000000000000000, 2.500000000000000000, -410.4979246179000256 ) ) ;
#9476=CARTESIAN_POINT ( 'NONE',  ( 14.00000000000000000, 2.500000000000000000, -272.5000000000000000 ) ) ;
#9483=LINE ( 'NONE', #4481, #5339 ) ;
#9490=( LENGTH_UNIT ( ) NAMED_UNIT ( * ) SI_UNIT ( .MILLI., .METRE. ) );
#9505=DIRECTION ( 'NONE',  ( 0.000000000000000000, -1.000000000000000000, 0.000000000000000000 ) ) ;
#9508=DIRECTION ( 'NONE',  ( 0.3420201433256988555, 0.000000000000000000, -0.9396926207858975477 ) ) ;
#9559=CARTESIAN_POINT ( 'NONE',  ( -38.59226537204000351, 2.500000000000000000, -500.7880554352000217 ) ) ;
#9560=CARTESIAN_POINT ( 'NONE',  ( -56.92031869107000119, -2.500000000000000000, -403.1217184488000385 ) ) ;
#9572=ORIENTED_EDGE ( 'NONE', *, *, #1807, .F. ) ;
#9584=DIRECTION ( 'NONE',  ( -0.3420201433256991330, 0.000000000000000000, 0.9396926207858973257 ) ) ;
#9597=ORIENTED_EDGE ( 'NONE', *, *, #1084, .F. ) ;
#9634=VERTEX_POINT ( 'NONE', #93 ) ;
#9647=CIRCLE ( 'NONE', #10324, 3.500000000000003109 ) ;
#9678=DIRECTION ( 'NONE',  ( 0.000000000000000000, -1.000000000000000000, 0.000000000000000000 ) ) ;
#9685=ORIENTED_EDGE ( 'NONE', *, *, #2068, .F. ) ;
#9698=ORIENTED_EDGE ( 'NONE', *, *, #5141, .F. ) ;
#9720=DIRECTION ( 'NONE',  ( -1.000000000000000000, 0.000000000000000000, 0.000000000000000000 ) ) ;
#9747=CARTESIAN_POINT ( 'NONE',  ( -14.00000000000000000, -2.500000000000000000, -317.5000000000000000 ) ) ;
#9765=CARTESIAN_POINT ( 'NONE',  ( -14.00000000000000000, -2.500000000000000000, -380.4979246178999688 ) ) ;
#9766=VERTEX_POINT ( 'NONE', #3581 ) ;
#9780=ORIENTED_EDGE ( 'NONE', *, *, #3202, .F. ) ;
#9793=LINE ( 'NONE', #1572, #9127 ) ;
#9807=DIRECTION ( 'NONE',  ( 0.000000000000000000, -1.000000000000000000, 0.000000000000000000 ) ) ;
#9828=AXIS2_PLACEMENT_3D ( 'NONE', #3322, #1872, #6767 ) ;
#9838=ADVANCED_FACE ( 'NONE', ( #2227 ), #6251, .T. ) ;
#9848=ORIENTED_EDGE ( 'NONE', *, *, #113, .F. ) ;
#9850=DIRECTION ( 'NONE',  ( -0.9396926207858972147, 0.000000000000000000, -0.3420201433256990775 ) ) ;
#9854=VECTOR ( 'NONE', #2234, 1000.000000000000000 ) ;
#9880=EDGE_CURVE ( 'NONE', #4852, #9887, #6468, .T. ) ;
#9887=VERTEX_POINT ( 'NONE', #2337 ) ;
#9897=ORIENTED_EDGE ( 'NONE', *, *, #4829, .T. ) ;
#9901=CARTESIAN_POINT ( 'NONE',  ( -2.000000000000000000, 2.500000000000000000, -409.5000000000000568 ) ) ;
#9912=CARTESIAN_POINT ( 'NONE',  ( -14.00000000000000000, 2.500000000000000000, -380.4979246178999688 ) ) ;
#9932=CYLINDRICAL_SURFACE ( 'NONE', #9828, 10.00000000000000000 ) ;
#9953=DIRECTION ( 'NONE',  ( 0.000000000000000000, -1.000000000000000000, 0.000000000000000000 ) ) ;
#9961=EDGE_CURVE ( 'NONE', #4332, #2247, #4322, .T. ) ;
#9991=ORIENTED_EDGE ( 'NONE', *, *, #9047, .T. ) ;
#9992=CARTESIAN_POINT ( 'NONE',  ( -17.18550143358999449, 2.500000000000000000, -495.8459145668000474 ) ) ;
#9994=ORIENTED_EDGE ( 'NONE', *, *, #2679, .T. ) ;
#10006=VECTOR ( 'NONE', #1385, 1000.000000000000000 ) ;
#10027=ORIENTED_EDGE ( 'NONE', *, *, #8494, .T. ) ;
#10038=VECTOR ( 'NONE', #5244, 1000.000000000000000 ) ;
#10067=ORIENTED_EDGE ( 'NONE', *, *, #2610, .T. ) ;
#10068=CARTESIAN_POINT ( 'NONE',  ( 14.00000000000000000, -2.500000000000000000, -317.5000000000000000 ) ) ;
#10083=EDGE_LOOP ( 'NONE', ( #5659, #7982, #3839, #4248 ) ) ;
#10120=ORIENTED_EDGE ( 'NONE', *, *, #6931, .F. ) ;
#10127=CARTESIAN_POINT ( 'NONE',  ( -38.59226537204000351, -2.500000000000000000, -500.7880554352000217 ) ) ;
#10128=ORIENTED_EDGE ( 'NONE', *, *, #114, .F. ) ;
#10138=MECHANICAL_DESIGN_GEOMETRIC_PRESENTATION_REPRESENTATION('',(#4138),#9290);
#10142=DIRECTION ( 'NONE',  ( 0.000000000000000000, -1.000000000000000000, 0.000000000000000000 ) ) ;
#10158=CIRCLE ( 'NONE', #9467, 10.00000000000000533 ) ;
#10160=DIRECTION ( 'NONE',  ( -0.000000000000000000, 1.000000000000000000, 0.000000000000000000 ) ) ;
#10161=EDGE_CURVE ( 'NONE', #2769, #8773, #1918, .T. ) ;
#10162=CARTESIAN_POINT ( 'NONE',  ( -50.24071243418999444, 2.500000000000000000, -414.3237589990000629 ) ) ;
#10174=EDGE_CURVE ( 'NONE', #886, #8632, #5190, .T. ) ;
#10181=DIRECTION ( 'NONE',  ( 0.000000000000000000, 1.000000000000000000, 0.000000000000000000 ) ) ;
#10184=VECTOR ( 'NONE', #6413, 1000.000000000000000 ) ;
#10205=AXIS2_PLACEMENT_3D ( 'NONE', #8984, #2534, #2589 ) ;
#10214=LINE ( 'NONE', #2851, #6078 ) ;
#10217=DIRECTION ( 'NONE',  ( -0.9612616959383172288, 0.000000000000000000, -0.2756373558170051030 ) ) ;
#10257=CARTESIAN_POINT ( 'NONE',  ( -14.00000000000000000, -2.500000000000000000, -317.5000000000000000 ) ) ;
#10263=CARTESIAN_POINT ( 'NONE',  ( -28.01838671672000203, 2.500000000000000000, -497.7560445212000104 ) ) ;
#10268=CARTESIAN_POINT ( 'NONE',  ( -28.01838671672000203, -2.500000000000000000, -497.7560445212000104 ) ) ;
#10270=ORIENTED_EDGE ( 'NONE', *, *, #9880, .F. ) ;
#10286=ORIENTED_EDGE ( 'NONE', *, *, #1003, .F. ) ;
#10310=DIRECTION ( 'NONE',  ( 0.000000000000000000, 1.000000000000000000, 0.000000000000000000 ) ) ;
#10324=AXIS2_PLACEMENT_3D ( 'NONE', #9193, #7517, #3435 ) ;
#10328=ORIENTED_EDGE ( 'NONE', *, *, #5932, .T. ) ;
#10372=CIRCLE ( 'NONE', #1111, 11.00000000000000000 ) ;
#10379=SURFACE_SIDE_STYLE ('',( #3019 ) ) ;
#10404=VERTEX_POINT ( 'NONE', #6971 ) ;
#10410=FACE_OUTER_BOUND ( 'NONE', #1359, .T. ) ;
#10428=CARTESIAN_POINT ( 'NONE',  ( -10.00000000000000000, 2.500000000000000000, -272.5000000000000000 ) ) ;
#10448=( NAMED_UNIT ( * ) SI_UNIT ( $, .STERADIAN. ) SOLID_ANGLE_UNIT ( ) );
#10456=VERTEX_POINT ( 'NONE', #3635 ) ;
#10474=DIRECTION ( 'NONE',  ( 0.000000000000000000, 0.000000000000000000, 1.000000000000000000 ) ) ;
#10483=( NAMED_UNIT ( * ) PLANE_ANGLE_UNIT ( ) SI_UNIT ( $, .RADIAN. ) );
#10491=LINE ( 'NONE', #3833, #7601 ) ;
#10497=ORIENTED_EDGE ( 'NONE', *, *, #6872, .F. ) ;
#10510=VECTOR ( 'NONE', #8318, 1000.000000000000000 ) ;
#10522=ORIENTED_EDGE ( 'NONE', *, *, #9040, .T. ) ;
#10529=DIRECTION ( 'NONE',  ( 0.000000000000000000, -1.000000000000000000, 0.000000000000000000 ) ) ;
#10570=ORIENTED_EDGE ( 'NONE', *, *, #3707, .F. ) ;
#10573=CARTESIAN_POINT ( 'NONE',  ( -2.000000000000000000, -2.500000000000000000, -409.5000000000000568 ) ) ;
#10581=ORIENTED_EDGE ( 'NONE', *, *, #5233, .F. ) ;
#10609=ADVANCED_FACE ( 'NONE', ( #10410 ), #3806, .T. ) ;
ENDSEC;
END-ISO-10303-21;
